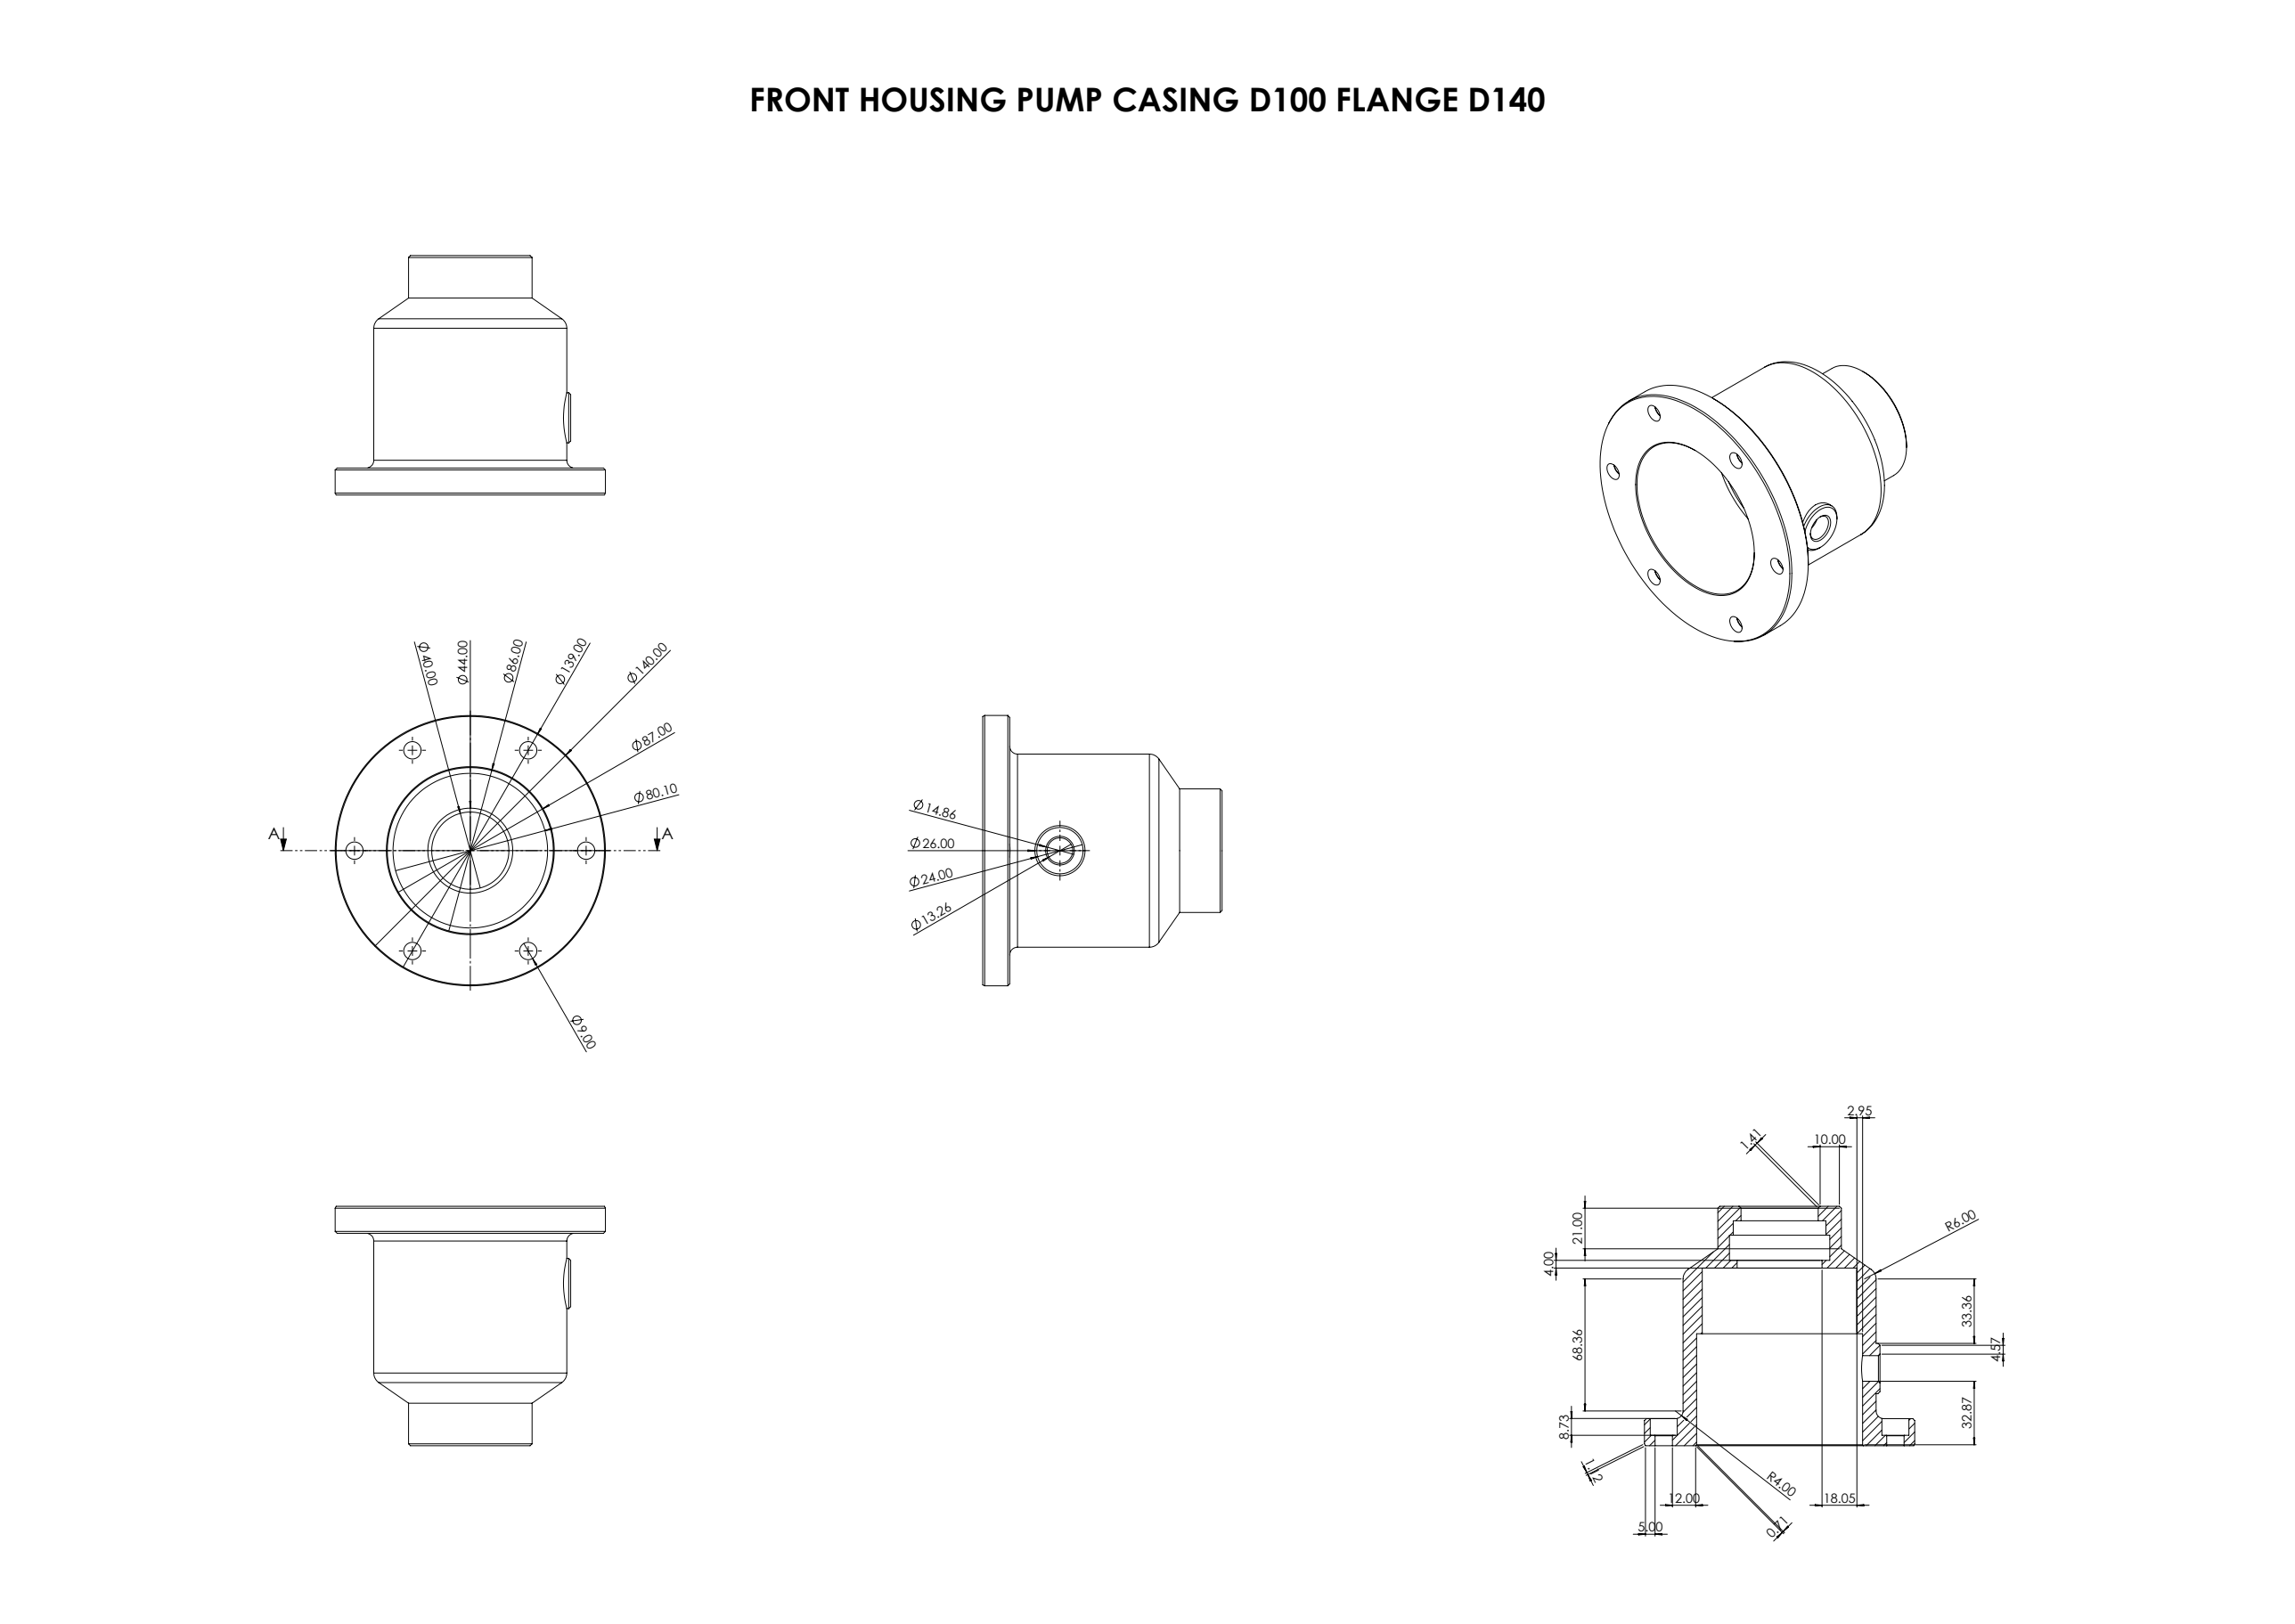
ISO-10303-21;
HEADER;
/* Generated by software containing ST-Developer
 * from STEP Tools, Inc. (www.steptools.com) 
 */

FILE_DESCRIPTION(
/* description */ (''),
/* implementation_level */ '2;1');

FILE_NAME(
/* name */ '01_Front_Housing_Pump_Casing_D100_Flange_D140.step',
/* time_stamp */ '2026-10-23T00:52:27+05:00',
/* author */ (''),
/* organization */ (''),
/* preprocessor_version */ 'ST-DEVELOPER v20.2',
/* originating_system */ 'Autodesk Translation Framework v15.15.0.0',
/* authorisation */ '');

FILE_SCHEMA (('AUTOMOTIVE_DESIGN { 1 0 10303 214 3 1 1 }'));
ENDSEC;

DATA;
#10=MECHANICAL_DESIGN_GEOMETRIC_PRESENTATION_REPRESENTATION('',(#1558,#1559,#1560,#1561,#1562,#1563,#1564),#59204);
#310=TOROIDAL_SURFACE('',#23784,5.4,0.4);
#311=TOROIDAL_SURFACE('',#23834,4.4,0.6);
#692=B_SPLINE_CURVE_WITH_KNOTS('',3,(#42442,#42443,#42444,#42445,#42446,
#42447,#42448,#42449,#42450,#42451,#42452,#42453,#42454,#42455,#42456,#42457),
 .UNSPECIFIED.,.F.,.F.,(4,2,2,2,2,2,2,4),(-0.827444006878981,-0.709137715093229,
-0.606258454477036,-0.552969769025734,-0.51054365769559,-0.463186805002842,
-0.385864633040324,-0.216479568668788),.UNSPECIFIED.);
#693=B_SPLINE_CURVE_WITH_KNOTS('',3,(#42466,#42467,#42468,#42469,#42470,
#42471,#42472,#42473,#42474,#42475),.UNSPECIFIED.,.F.,.F.,(4,2,2,2,4),(-0.52479568404363,
-0.512334893121172,-0.461457866065132,-0.380752711923638,-0.216468504749557),
 .UNSPECIFIED.);
#694=B_SPLINE_CURVE_WITH_KNOTS('',3,(#42479,#42480,#42481,#42482,#42483,
#42484,#42485,#42486,#42487,#42488,#42489,#42490,#42491,#42492,#42493,#42494),
 .UNSPECIFIED.,.F.,.F.,(4,2,2,2,2,2,2,4),(-0.827444006877975,-0.709137715092587,
-0.606258454476783,-0.552969769025578,-0.510543657695527,-0.463186805002854,
-0.385864633040295,-0.216479568668763),.UNSPECIFIED.);
#695=B_SPLINE_CURVE_WITH_KNOTS('',3,(#42498,#42499,#42500,#42501,#42502,
#42503,#42504,#42505,#42506,#42507,#42508,#42509,#42510,#42511,#42512,#42513),
 .UNSPECIFIED.,.F.,.F.,(4,2,2,2,2,2,2,4),(-0.827444006878145,-0.709137715092748,
-0.606258454476905,-0.552969769025703,-0.510543657695638,-0.463186805002939,
-0.385864633040348,-0.21647956866881),.UNSPECIFIED.);
#696=B_SPLINE_CURVE_WITH_KNOTS('',3,(#42517,#42518,#42519,#42520,#42521,
#42522,#42523,#42524,#42525,#42526),.UNSPECIFIED.,.F.,.F.,(4,2,2,2,4),(-0.828799355587065,
-0.7357048796955,-0.618324369294947,-0.558811967132771,-0.524795684044317),
 .UNSPECIFIED.);
#697=B_SPLINE_CURVE_WITH_KNOTS('',3,(#42528,#42529,#42530,#42531,#42532,
#42533,#42534,#42535,#42536,#42537),.UNSPECIFIED.,.F.,.F.,(4,2,2,2,4),(-0.524795684044317,
-0.512334893121834,-0.461457866065708,-0.380752711924124,-0.216468504749763),
 .UNSPECIFIED.);
#698=B_SPLINE_CURVE_WITH_KNOTS('',3,(#42542,#42543,#42544,#42545,#42546,
#42547,#42548,#42549,#42550,#42551,#42552,#42553,#42554,#42555,#42556,#42557),
 .UNSPECIFIED.,.F.,.F.,(4,2,2,2,2,2,2,4),(-0.827444006877793,-0.709137715092454,
-0.606258454476639,-0.552969769025454,-0.510543657695402,-0.463186805002724,
-0.385864633040191,-0.216479568668727),.UNSPECIFIED.);
#699=B_SPLINE_CURVE_WITH_KNOTS('',3,(#42560,#42561,#42562,#42563,#42564,
#42565,#42566,#42567,#42568,#42569),.UNSPECIFIED.,.F.,.F.,(4,2,2,2,4),(-0.828799355585381,
-0.735704879694107,-0.618324369293949,-0.558811967131987,-0.52479568404363),
 .UNSPECIFIED.);
#700=B_SPLINE_CURVE_WITH_KNOTS('',3,(#42606,#42607,#42608,#42609,#42610,
#42611,#42612,#42613,#42614,#42615),.UNSPECIFIED.,.F.,.F.,(4,2,2,2,4),(0.,
0.250118116648096,0.500236233296193,0.750349479868711,1.00046272644123),
 .UNSPECIFIED.);
#701=B_SPLINE_CURVE_WITH_KNOTS('',3,(#42616,#42617,#42618,#42619,#42620,
#42621,#42622,#42623,#42624,#42625,#42626,#42627,#42628,#42629,#42630,#42631,
#42632,#42633,#42634,#42635,#42636,#42637,#42638,#42639,#42640,#42641),
 .UNSPECIFIED.,.F.,.F.,(4,2,2,2,2,2,2,2,2,2,2,2,4),(1.00046272644123,1.25057597301375,
1.50068921958627,1.75080733623436,2.00092545288246,2.25104356953056,2.50116168617865,
2.75127493275117,3.00138817932369,3.25150142589621,3.50161467246873,3.75173278911682,
4.00185090576492),.UNSPECIFIED.);
#702=B_SPLINE_CURVE_WITH_KNOTS('',3,(#42653,#42654,#42655,#42656,#42657,
#42658,#42659,#42660,#42661,#42662,#42663,#42664,#42665,#42666,#42667,#42668,
#42669,#42670,#42671,#42672,#42673,#42674,#42675,#42676,#42677,#42678),
 .UNSPECIFIED.,.F.,.F.,(4,2,2,2,2,2,2,2,2,2,2,2,4),(0.,0.492179153056542,
0.984358306113084,1.47645655199157,1.96855479787006,2.46065304374855,2.95275128962704,
3.44493044268358,3.93710959574012,4.42928874879666,4.92146790185321,5.41356614773169,
5.90566439361018),.UNSPECIFIED.);
#703=B_SPLINE_CURVE_WITH_KNOTS('',3,(#42679,#42680,#42681,#42682,#42683,
#42684,#42685,#42686,#42687,#42688),.UNSPECIFIED.,.F.,.F.,(4,2,2,2,4),(5.90566439361018,
6.39776263948867,6.88986088536716,7.3820400384237,7.87421919148024),
 .UNSPECIFIED.);
#1518=SHAPE_REPRESENTATION_RELATIONSHIP('SRR','None',#59307,#1538);
#1538=ADVANCED_BREP_SHAPE_REPRESENTATION('',(#1585),#59194);
#1558=STYLED_ITEM('',(#59565),#21883);
#1559=STYLED_ITEM('',(#59565),#21884);
#1560=STYLED_ITEM('',(#59565),#21885);
#1561=STYLED_ITEM('',(#59565),#21908);
#1562=STYLED_ITEM('',(#59565),#21911);
#1563=STYLED_ITEM('',(#59565),#21915);
#1564=STYLED_ITEM('',(#59565),#1585);
#1585=MANIFOLD_SOLID_BREP('Front housing',#22814);
#1670=FACE_BOUND('',#4431,.T.);
#1671=FACE_BOUND('',#4435,.T.);
#1672=FACE_BOUND('',#4439,.T.);
#1673=FACE_BOUND('',#4443,.T.);
#1674=FACE_BOUND('',#4447,.T.);
#1675=FACE_BOUND('',#4451,.T.);
#1676=FACE_BOUND('',#4457,.T.);
#1677=FACE_BOUND('',#4465,.T.);
#1678=FACE_BOUND('',#4470,.T.);
#1679=FACE_BOUND('',#4471,.T.);
#1680=FACE_BOUND('',#4472,.T.);
#1681=FACE_BOUND('',#4473,.T.);
#1682=FACE_BOUND('',#4474,.T.);
#1683=FACE_BOUND('',#4475,.T.);
#1684=FACE_BOUND('',#4476,.T.);
#1685=FACE_BOUND('',#4478,.T.);
#1686=FACE_BOUND('',#4482,.T.);
#1687=FACE_BOUND('',#4483,.T.);
#1688=FACE_BOUND('',#4486,.T.);
#1689=FACE_BOUND('',#4494,.T.);
#1690=FACE_BOUND('',#4497,.T.);
#1691=FACE_BOUND('',#4500,.T.);
#1692=FACE_BOUND('',#4503,.T.);
#1693=FACE_BOUND('',#4506,.T.);
#2020=PLANE('',#23721);
#2021=PLANE('',#23722);
#2022=PLANE('',#23723);
#2023=PLANE('',#23724);
#2024=PLANE('',#23728);
#2025=PLANE('',#23732);
#2026=PLANE('',#23737);
#2027=PLANE('',#23745);
#2028=PLANE('',#23753);
#2029=PLANE('',#23761);
#2030=PLANE('',#23769);
#2031=PLANE('',#23777);
#2032=PLANE('',#23796);
#2033=PLANE('',#23813);
#2034=PLANE('',#23822);
#2035=PLANE('',#23832);
#2036=PLANE('',#23849);
#2037=PLANE('',#23853);
#2038=PLANE('',#23857);
#2039=PLANE('',#23861);
#2040=PLANE('',#23865);
#2504=CYLINDRICAL_SURFACE('',#23725,2.56);
#2505=CYLINDRICAL_SURFACE('',#23729,2.84);
#2506=CYLINDRICAL_SURFACE('',#23739,0.45);
#2507=CYLINDRICAL_SURFACE('',#23747,0.45);
#2508=CYLINDRICAL_SURFACE('',#23755,0.45);
#2509=CYLINDRICAL_SURFACE('',#23763,0.45);
#2510=CYLINDRICAL_SURFACE('',#23771,0.45);
#2511=CYLINDRICAL_SURFACE('',#23779,0.45);
#2512=CYLINDRICAL_SURFACE('',#23781,0.7);
#2513=CYLINDRICAL_SURFACE('',#23793,0.7);
#2514=CYLINDRICAL_SURFACE('',#23805,0.7);
#2515=CYLINDRICAL_SURFACE('',#23806,0.7);
#2516=CYLINDRICAL_SURFACE('',#23807,0.7);
#2517=CYLINDRICAL_SURFACE('',#23808,0.7);
#2518=CYLINDRICAL_SURFACE('',#23812,0.66285);
#2519=CYLINDRICAL_SURFACE('',#23817,1.3);
#2520=CYLINDRICAL_SURFACE('',#23824,4.3);
#2521=CYLINDRICAL_SURFACE('',#23830,2.);
#2522=CYLINDRICAL_SURFACE('',#23838,5.);
#2523=CYLINDRICAL_SURFACE('',#23843,3.2);
#2524=CYLINDRICAL_SURFACE('',#23846,7.);
#2525=CYLINDRICAL_SURFACE('',#23851,4.005);
#2526=CYLINDRICAL_SURFACE('',#23855,2.2);
#2527=CYLINDRICAL_SURFACE('',#23859,2.6);
#2528=CYLINDRICAL_SURFACE('',#23863,2.4);
#3045=FACE_OUTER_BOUND('',#4421,.T.);
#3046=FACE_OUTER_BOUND('',#4422,.T.);
#3047=FACE_OUTER_BOUND('',#4423,.T.);
#3048=FACE_OUTER_BOUND('',#4424,.T.);
#3049=FACE_OUTER_BOUND('',#4425,.T.);
#3050=FACE_OUTER_BOUND('',#4426,.T.);
#3051=FACE_OUTER_BOUND('',#4427,.T.);
#3052=FACE_OUTER_BOUND('',#4428,.T.);
#3053=FACE_OUTER_BOUND('',#4429,.T.);
#3054=FACE_OUTER_BOUND('',#4430,.T.);
#3055=FACE_OUTER_BOUND('',#4432,.T.);
#3056=FACE_OUTER_BOUND('',#4433,.T.);
#3057=FACE_OUTER_BOUND('',#4434,.T.);
#3058=FACE_OUTER_BOUND('',#4436,.T.);
#3059=FACE_OUTER_BOUND('',#4437,.T.);
#3060=FACE_OUTER_BOUND('',#4438,.T.);
#3061=FACE_OUTER_BOUND('',#4440,.T.);
#3062=FACE_OUTER_BOUND('',#4441,.T.);
#3063=FACE_OUTER_BOUND('',#4442,.T.);
#3064=FACE_OUTER_BOUND('',#4444,.T.);
#3065=FACE_OUTER_BOUND('',#4445,.T.);
#3066=FACE_OUTER_BOUND('',#4446,.T.);
#3067=FACE_OUTER_BOUND('',#4448,.T.);
#3068=FACE_OUTER_BOUND('',#4449,.T.);
#3069=FACE_OUTER_BOUND('',#4450,.T.);
#3070=FACE_OUTER_BOUND('',#4452,.T.);
#3071=FACE_OUTER_BOUND('',#4453,.T.);
#3072=FACE_OUTER_BOUND('',#4454,.T.);
#3073=FACE_OUTER_BOUND('',#4455,.T.);
#3074=FACE_OUTER_BOUND('',#4456,.T.);
#3075=FACE_OUTER_BOUND('',#4458,.T.);
#3076=FACE_OUTER_BOUND('',#4459,.T.);
#3077=FACE_OUTER_BOUND('',#4460,.T.);
#3078=FACE_OUTER_BOUND('',#4461,.T.);
#3079=FACE_OUTER_BOUND('',#4462,.T.);
#3080=FACE_OUTER_BOUND('',#4463,.T.);
#3081=FACE_OUTER_BOUND('',#4464,.T.);
#3082=FACE_OUTER_BOUND('',#4466,.T.);
#3083=FACE_OUTER_BOUND('',#4467,.T.);
#3084=FACE_OUTER_BOUND('',#4468,.T.);
#3085=FACE_OUTER_BOUND('',#4469,.T.);
#3086=FACE_OUTER_BOUND('',#4477,.T.);
#3087=FACE_OUTER_BOUND('',#4479,.T.);
#3088=FACE_OUTER_BOUND('',#4480,.T.);
#3089=FACE_OUTER_BOUND('',#4481,.T.);
#3090=FACE_OUTER_BOUND('',#4484,.T.);
#3091=FACE_OUTER_BOUND('',#4485,.T.);
#3092=FACE_OUTER_BOUND('',#4487,.T.);
#3093=FACE_OUTER_BOUND('',#4488,.T.);
#3094=FACE_OUTER_BOUND('',#4489,.T.);
#3095=FACE_OUTER_BOUND('',#4490,.T.);
#3096=FACE_OUTER_BOUND('',#4491,.T.);
#3097=FACE_OUTER_BOUND('',#4492,.T.);
#3098=FACE_OUTER_BOUND('',#4493,.T.);
#3099=FACE_OUTER_BOUND('',#4495,.T.);
#3100=FACE_OUTER_BOUND('',#4496,.T.);
#3101=FACE_OUTER_BOUND('',#4498,.T.);
#3102=FACE_OUTER_BOUND('',#4499,.T.);
#3103=FACE_OUTER_BOUND('',#4501,.T.);
#3104=FACE_OUTER_BOUND('',#4502,.T.);
#3105=FACE_OUTER_BOUND('',#4504,.T.);
#3106=FACE_OUTER_BOUND('',#4505,.T.);
#4421=EDGE_LOOP('',(#16438,#16439,#16440,#16441));
#4422=EDGE_LOOP('',(#16442,#16443,#16444,#16445));
#4423=EDGE_LOOP('',(#16446,#16447,#16448,#16449));
#4424=EDGE_LOOP('',(#16450,#16451,#16452,#16453));
#4425=EDGE_LOOP('',(#16454,#16455,#16456,#16457));
#4426=EDGE_LOOP('',(#16458,#16459,#16460,#16461));
#4427=EDGE_LOOP('',(#16462,#16463,#16464,#16465));
#4428=EDGE_LOOP('',(#16466,#16467,#16468,#16469,#16470,#16471,#16472));
#4429=EDGE_LOOP('',(#16473,#16474,#16475,#16476,#16477));
#4430=EDGE_LOOP('',(#16478));
#4431=EDGE_LOOP('',(#16479));
#4432=EDGE_LOOP('',(#16480,#16481,#16482,#16483,#16484));
#4433=EDGE_LOOP('',(#16485,#16486,#16487,#16488,#16489));
#4434=EDGE_LOOP('',(#16490));
#4435=EDGE_LOOP('',(#16491));
#4436=EDGE_LOOP('',(#16492,#16493,#16494,#16495,#16496));
#4437=EDGE_LOOP('',(#16497,#16498,#16499,#16500,#16501));
#4438=EDGE_LOOP('',(#16502));
#4439=EDGE_LOOP('',(#16503));
#4440=EDGE_LOOP('',(#16504,#16505,#16506,#16507,#16508));
#4441=EDGE_LOOP('',(#16509,#16510,#16511,#16512,#16513));
#4442=EDGE_LOOP('',(#16514));
#4443=EDGE_LOOP('',(#16515));
#4444=EDGE_LOOP('',(#16516,#16517,#16518,#16519,#16520));
#4445=EDGE_LOOP('',(#16521,#16522,#16523,#16524,#16525));
#4446=EDGE_LOOP('',(#16526));
#4447=EDGE_LOOP('',(#16527));
#4448=EDGE_LOOP('',(#16528,#16529,#16530,#16531,#16532));
#4449=EDGE_LOOP('',(#16533,#16534,#16535,#16536,#16537));
#4450=EDGE_LOOP('',(#16538));
#4451=EDGE_LOOP('',(#16539));
#4452=EDGE_LOOP('',(#16540,#16541,#16542,#16543,#16544));
#4453=EDGE_LOOP('',(#16545,#16546,#16547,#16548,#16549,#16550));
#4454=EDGE_LOOP('',(#16551,#16552,#16553,#16554,#16555,#16556,#16557,#16558,
#16559,#16560,#16561,#16562,#16563,#16564,#16565,#16566,#16567));
#4455=EDGE_LOOP('',(#16568,#16569,#16570,#16571,#16572,#16573));
#4456=EDGE_LOOP('',(#16574));
#4457=EDGE_LOOP('',(#16575,#16576,#16577,#16578,#16579,#16580,#16581,#16582,
#16583,#16584,#16585,#16586,#16587,#16588,#16589,#16590,#16591));
#4458=EDGE_LOOP('',(#16592,#16593,#16594,#16595,#16596,#16597,#16598));
#4459=EDGE_LOOP('',(#16599,#16600,#16601,#16602,#16603,#16604));
#4460=EDGE_LOOP('',(#16605,#16606,#16607,#16608,#16609,#16610));
#4461=EDGE_LOOP('',(#16611,#16612,#16613,#16614,#16615,#16616));
#4462=EDGE_LOOP('',(#16617,#16618,#16619,#16620));
#4463=EDGE_LOOP('',(#16621,#16622,#16623,#16624,#16625));
#4464=EDGE_LOOP('',(#16626));
#4465=EDGE_LOOP('',(#16627));
#4466=EDGE_LOOP('',(#16628,#16629,#16630,#16631));
#4467=EDGE_LOOP('',(#16632,#16633,#16634,#16635,#16636));
#4468=EDGE_LOOP('',(#16637,#16638,#16639,#16640,#16641));
#4469=EDGE_LOOP('',(#16642));
#4470=EDGE_LOOP('',(#16643));
#4471=EDGE_LOOP('',(#16644));
#4472=EDGE_LOOP('',(#16645));
#4473=EDGE_LOOP('',(#16646));
#4474=EDGE_LOOP('',(#16647));
#4475=EDGE_LOOP('',(#16648));
#4476=EDGE_LOOP('',(#16649));
#4477=EDGE_LOOP('',(#16650,#16651,#16652,#16653,#16654));
#4478=EDGE_LOOP('',(#16655,#16656));
#4479=EDGE_LOOP('',(#16657,#16658,#16659,#16660,#16661));
#4480=EDGE_LOOP('',(#16662,#16663,#16664,#16665,#16666));
#4481=EDGE_LOOP('',(#16667));
#4482=EDGE_LOOP('',(#16668,#16669,#16670,#16671,#16672,#16673,#16674));
#4483=EDGE_LOOP('',(#16675));
#4484=EDGE_LOOP('',(#16676,#16677,#16678,#16679));
#4485=EDGE_LOOP('',(#16680,#16681,#16682,#16683));
#4486=EDGE_LOOP('',(#16684,#16685));
#4487=EDGE_LOOP('',(#16686,#16687,#16688,#16689));
#4488=EDGE_LOOP('',(#16690,#16691,#16692,#16693));
#4489=EDGE_LOOP('',(#16694,#16695,#16696,#16697));
#4490=EDGE_LOOP('',(#16698,#16699,#16700,#16701));
#4491=EDGE_LOOP('',(#16702,#16703,#16704,#16705));
#4492=EDGE_LOOP('',(#16706,#16707,#16708,#16709));
#4493=EDGE_LOOP('',(#16710));
#4494=EDGE_LOOP('',(#16711));
#4495=EDGE_LOOP('',(#16712,#16713,#16714,#16715));
#4496=EDGE_LOOP('',(#16716));
#4497=EDGE_LOOP('',(#16717));
#4498=EDGE_LOOP('',(#16718,#16719,#16720,#16721));
#4499=EDGE_LOOP('',(#16722));
#4500=EDGE_LOOP('',(#16723));
#4501=EDGE_LOOP('',(#16724,#16725,#16726,#16727));
#4502=EDGE_LOOP('',(#16728));
#4503=EDGE_LOOP('',(#16729));
#4504=EDGE_LOOP('',(#16730,#16731,#16732,#16733));
#4505=EDGE_LOOP('',(#16734));
#4506=EDGE_LOOP('',(#16735));
#5919=LINE('',#42307,#7352);
#5920=LINE('',#42309,#7353);
#5921=LINE('',#42311,#7354);
#5922=LINE('',#42312,#7355);
#5923=LINE('',#42315,#7356);
#5924=LINE('',#42317,#7357);
#5925=LINE('',#42318,#7358);
#5926=LINE('',#42321,#7359);
#5927=LINE('',#42323,#7360);
#5928=LINE('',#42324,#7361);
#5929=LINE('',#42327,#7362);
#5930=LINE('',#42329,#7363);
#5931=LINE('',#42330,#7364);
#5932=LINE('',#42335,#7365);
#5933=LINE('',#42339,#7366);
#5934=LINE('',#42341,#7367);
#5935=LINE('',#42342,#7368);
#5936=LINE('',#42351,#7369);
#5937=LINE('',#42360,#7370);
#5938=LINE('',#42366,#7371);
#5939=LINE('',#42375,#7372);
#5940=LINE('',#42381,#7373);
#5941=LINE('',#42390,#7374);
#5942=LINE('',#42396,#7375);
#5943=LINE('',#42405,#7376);
#5944=LINE('',#42411,#7377);
#5945=LINE('',#42420,#7378);
#5946=LINE('',#42426,#7379);
#5947=LINE('',#42435,#7380);
#5948=LINE('',#42459,#7381);
#5949=LINE('',#42573,#7382);
#5950=LINE('',#42589,#7383);
#5951=LINE('',#42591,#7384);
#5952=LINE('',#42593,#7385);
#5953=LINE('',#42595,#7386);
#5954=LINE('',#42600,#7387);
#5955=LINE('',#42604,#7388);
#5956=LINE('',#42647,#7389);
#5957=LINE('',#42651,#7390);
#5958=LINE('',#42695,#7391);
#5959=LINE('',#42702,#7392);
#5960=LINE('',#42708,#7393);
#5961=LINE('',#42715,#7394);
#5962=LINE('',#42726,#7395);
#5963=LINE('',#42729,#7396);
#5964=LINE('',#42734,#7397);
#5965=LINE('',#42736,#7398);
#5966=LINE('',#42740,#7399);
#5967=LINE('',#42744,#7400);
#5968=LINE('',#42746,#7401);
#5969=LINE('',#42752,#7402);
#5970=LINE('',#42759,#7403);
#5971=LINE('',#42766,#7404);
#5972=LINE('',#42773,#7405);
#7352=VECTOR('',#26899,1.);
#7353=VECTOR('',#26900,1.);
#7354=VECTOR('',#26901,1.);
#7355=VECTOR('',#26902,1.);
#7356=VECTOR('',#26905,1.);
#7357=VECTOR('',#26906,1.);
#7358=VECTOR('',#26907,1.);
#7359=VECTOR('',#26910,1.);
#7360=VECTOR('',#26911,1.);
#7361=VECTOR('',#26912,1.);
#7362=VECTOR('',#26915,1.);
#7363=VECTOR('',#26916,1.);
#7364=VECTOR('',#26917,1.);
#7365=VECTOR('',#26922,1.);
#7366=VECTOR('',#26927,1.);
#7367=VECTOR('',#26928,1.);
#7368=VECTOR('',#26929,1.);
#7369=VECTOR('',#26942,0.4625);
#7370=VECTOR('',#26953,0.45);
#7371=VECTOR('',#26960,0.4625);
#7372=VECTOR('',#26971,0.45);
#7373=VECTOR('',#26978,0.4625);
#7374=VECTOR('',#26989,0.45);
#7375=VECTOR('',#26996,0.4625);
#7376=VECTOR('',#27007,0.45);
#7377=VECTOR('',#27014,0.4625);
#7378=VECTOR('',#27025,0.45);
#7379=VECTOR('',#27032,0.4625);
#7380=VECTOR('',#27043,0.45);
#7381=VECTOR('',#27052,0.7);
#7382=VECTOR('',#27075,0.7);
#7383=VECTOR('',#27098,0.7);
#7384=VECTOR('',#27101,0.7);
#7385=VECTOR('',#27104,0.7);
#7386=VECTOR('',#27107,0.7);
#7387=VECTOR('',#27112,0.70285);
#7388=VECTOR('',#27117,0.66285);
#7389=VECTOR('',#27124,1.25);
#7390=VECTOR('',#27129,1.3);
#7391=VECTOR('',#27136,4.325);
#7392=VECTOR('',#27145,4.3);
#7393=VECTOR('',#27152,2.05);
#7394=VECTOR('',#27161,2.);
#7395=VECTOR('',#27176,5.);
#7396=VECTOR('',#27179,4.1);
#7397=VECTOR('',#27186,3.15);
#7398=VECTOR('',#27189,3.2);
#7399=VECTOR('',#27194,6.95);
#7400=VECTOR('',#27199,7.);
#7401=VECTOR('',#27202,6.975);
#7402=VECTOR('',#27209,4.005);
#7403=VECTOR('',#27218,2.2);
#7404=VECTOR('',#27227,2.6);
#7405=VECTOR('',#27236,2.4);
#8662=CIRCLE('',#23726,2.56);
#8663=CIRCLE('',#23727,2.56);
#8664=CIRCLE('',#23730,2.84);
#8665=CIRCLE('',#23731,2.84);
#8666=CIRCLE('',#23734,0.475000000000001);
#8667=CIRCLE('',#23735,0.45);
#8668=CIRCLE('',#23736,0.45);
#8669=CIRCLE('',#23738,0.7);
#8670=CIRCLE('',#23740,0.45);
#8671=CIRCLE('',#23742,0.475);
#8672=CIRCLE('',#23743,0.45);
#8673=CIRCLE('',#23744,0.45);
#8674=CIRCLE('',#23746,0.7);
#8675=CIRCLE('',#23748,0.45);
#8676=CIRCLE('',#23750,0.475);
#8677=CIRCLE('',#23751,0.45);
#8678=CIRCLE('',#23752,0.45);
#8679=CIRCLE('',#23754,0.7);
#8680=CIRCLE('',#23756,0.45);
#8681=CIRCLE('',#23758,0.475000000000001);
#8682=CIRCLE('',#23759,0.45);
#8683=CIRCLE('',#23760,0.45);
#8684=CIRCLE('',#23762,0.7);
#8685=CIRCLE('',#23764,0.45);
#8686=CIRCLE('',#23766,0.475);
#8687=CIRCLE('',#23767,0.45);
#8688=CIRCLE('',#23768,0.45);
#8689=CIRCLE('',#23770,0.7);
#8690=CIRCLE('',#23772,0.45);
#8691=CIRCLE('',#23774,0.475);
#8692=CIRCLE('',#23775,0.45);
#8693=CIRCLE('',#23776,0.45);
#8694=CIRCLE('',#23778,0.7);
#8695=CIRCLE('',#23780,0.45);
#8696=CIRCLE('',#23782,0.7);
#8697=CIRCLE('',#23783,0.7);
#8698=CIRCLE('',#23785,5.);
#8699=CIRCLE('',#23786,0.4);
#8700=CIRCLE('',#23787,5.4);
#8701=CIRCLE('',#23788,5.4);
#8702=CIRCLE('',#23789,5.4);
#8703=CIRCLE('',#23790,5.4);
#8704=CIRCLE('',#23791,5.4);
#8705=CIRCLE('',#23792,5.4);
#8706=CIRCLE('',#23794,0.7);
#8707=CIRCLE('',#23795,0.7);
#8708=CIRCLE('',#23797,6.9);
#8709=CIRCLE('',#23798,0.7);
#8710=CIRCLE('',#23799,0.7);
#8711=CIRCLE('',#23800,0.7);
#8712=CIRCLE('',#23801,0.7);
#8713=CIRCLE('',#23802,0.7);
#8714=CIRCLE('',#23803,0.7);
#8715=CIRCLE('',#23804,0.7);
#8716=CIRCLE('',#23810,0.74285);
#8717=CIRCLE('',#23811,0.66285);
#8718=CIRCLE('',#23814,1.2);
#8719=CIRCLE('',#23816,1.3);
#8720=CIRCLE('',#23819,4.3);
#8721=CIRCLE('',#23820,4.3);
#8722=CIRCLE('',#23821,4.35);
#8723=CIRCLE('',#23823,6.95);
#8724=CIRCLE('',#23825,4.3);
#8725=CIRCLE('',#23827,2.1);
#8726=CIRCLE('',#23828,2.);
#8727=CIRCLE('',#23829,2.);
#8728=CIRCLE('',#23831,2.);
#8729=CIRCLE('',#23833,3.1);
#8730=CIRCLE('',#23835,5.);
#8731=CIRCLE('',#23836,0.6);
#8732=CIRCLE('',#23837,4.74223748569721);
#8733=CIRCLE('',#23840,3.2);
#8734=CIRCLE('',#23842,3.2);
#8735=CIRCLE('',#23845,7.);
#8736=CIRCLE('',#23847,7.);
#8737=CIRCLE('',#23850,4.005);
#8738=CIRCLE('',#23852,4.005);
#8739=CIRCLE('',#23854,2.2);
#8740=CIRCLE('',#23856,2.2);
#8741=CIRCLE('',#23858,2.6);
#8742=CIRCLE('',#23860,2.6);
#8743=CIRCLE('',#23862,2.4);
#8744=CIRCLE('',#23864,2.4);
#9749=VERTEX_POINT('',#42305);
#9750=VERTEX_POINT('',#42306);
#9751=VERTEX_POINT('',#42308);
#9752=VERTEX_POINT('',#42310);
#9753=VERTEX_POINT('',#42314);
#9754=VERTEX_POINT('',#42316);
#9755=VERTEX_POINT('',#42320);
#9756=VERTEX_POINT('',#42322);
#9757=VERTEX_POINT('',#42326);
#9758=VERTEX_POINT('',#42328);
#9759=VERTEX_POINT('',#42332);
#9760=VERTEX_POINT('',#42334);
#9761=VERTEX_POINT('',#42338);
#9762=VERTEX_POINT('',#42340);
#9763=VERTEX_POINT('',#42348);
#9764=VERTEX_POINT('',#42350);
#9765=VERTEX_POINT('',#42352);
#9766=VERTEX_POINT('',#42356);
#9767=VERTEX_POINT('',#42359);
#9768=VERTEX_POINT('',#42363);
#9769=VERTEX_POINT('',#42365);
#9770=VERTEX_POINT('',#42367);
#9771=VERTEX_POINT('',#42371);
#9772=VERTEX_POINT('',#42374);
#9773=VERTEX_POINT('',#42378);
#9774=VERTEX_POINT('',#42380);
#9775=VERTEX_POINT('',#42382);
#9776=VERTEX_POINT('',#42386);
#9777=VERTEX_POINT('',#42389);
#9778=VERTEX_POINT('',#42393);
#9779=VERTEX_POINT('',#42395);
#9780=VERTEX_POINT('',#42397);
#9781=VERTEX_POINT('',#42401);
#9782=VERTEX_POINT('',#42404);
#9783=VERTEX_POINT('',#42408);
#9784=VERTEX_POINT('',#42410);
#9785=VERTEX_POINT('',#42412);
#9786=VERTEX_POINT('',#42416);
#9787=VERTEX_POINT('',#42419);
#9788=VERTEX_POINT('',#42423);
#9789=VERTEX_POINT('',#42425);
#9790=VERTEX_POINT('',#42427);
#9791=VERTEX_POINT('',#42431);
#9792=VERTEX_POINT('',#42434);
#9793=VERTEX_POINT('',#42438);
#9794=VERTEX_POINT('',#42439);
#9795=VERTEX_POINT('',#42441);
#9796=VERTEX_POINT('',#42461);
#9797=VERTEX_POINT('',#42463);
#9798=VERTEX_POINT('',#42465);
#9799=VERTEX_POINT('',#42476);
#9800=VERTEX_POINT('',#42478);
#9801=VERTEX_POINT('',#42495);
#9802=VERTEX_POINT('',#42497);
#9803=VERTEX_POINT('',#42514);
#9804=VERTEX_POINT('',#42516);
#9805=VERTEX_POINT('',#42527);
#9806=VERTEX_POINT('',#42539);
#9807=VERTEX_POINT('',#42541);
#9808=VERTEX_POINT('',#42558);
#9809=VERTEX_POINT('',#42571);
#9810=VERTEX_POINT('',#42576);
#9811=VERTEX_POINT('',#42579);
#9812=VERTEX_POINT('',#42582);
#9813=VERTEX_POINT('',#42585);
#9814=VERTEX_POINT('',#42597);
#9815=VERTEX_POINT('',#42599);
#9816=VERTEX_POINT('',#42603);
#9817=VERTEX_POINT('',#42605);
#9818=VERTEX_POINT('',#42643);
#9819=VERTEX_POINT('',#42646);
#9820=VERTEX_POINT('',#42650);
#9821=VERTEX_POINT('',#42652);
#9822=VERTEX_POINT('',#42690);
#9823=VERTEX_POINT('',#42691);
#9824=VERTEX_POINT('',#42694);
#9825=VERTEX_POINT('',#42698);
#9826=VERTEX_POINT('',#42701);
#9827=VERTEX_POINT('',#42705);
#9828=VERTEX_POINT('',#42707);
#9829=VERTEX_POINT('',#42709);
#9830=VERTEX_POINT('',#42713);
#9831=VERTEX_POINT('',#42717);
#9832=VERTEX_POINT('',#42720);
#9833=VERTEX_POINT('',#42722);
#9834=VERTEX_POINT('',#42728);
#9835=VERTEX_POINT('',#42732);
#9836=VERTEX_POINT('',#42738);
#9837=VERTEX_POINT('',#42742);
#9838=VERTEX_POINT('',#42748);
#9839=VERTEX_POINT('',#42751);
#9840=VERTEX_POINT('',#42755);
#9841=VERTEX_POINT('',#42758);
#9842=VERTEX_POINT('',#42762);
#9843=VERTEX_POINT('',#42765);
#9844=VERTEX_POINT('',#42769);
#9845=VERTEX_POINT('',#42772);
#12223=EDGE_CURVE('',#9749,#9750,#5919,.T.);
#12224=EDGE_CURVE('',#9749,#9751,#5920,.T.);
#12225=EDGE_CURVE('',#9751,#9752,#5921,.T.);
#12226=EDGE_CURVE('',#9750,#9752,#5922,.T.);
#12227=EDGE_CURVE('',#9753,#9749,#5923,.T.);
#12228=EDGE_CURVE('',#9753,#9754,#5924,.T.);
#12229=EDGE_CURVE('',#9754,#9751,#5925,.T.);
#12230=EDGE_CURVE('',#9755,#9753,#5926,.T.);
#12231=EDGE_CURVE('',#9755,#9756,#5927,.T.);
#12232=EDGE_CURVE('',#9756,#9754,#5928,.T.);
#12233=EDGE_CURVE('',#9757,#9755,#5929,.T.);
#12234=EDGE_CURVE('',#9757,#9758,#5930,.T.);
#12235=EDGE_CURVE('',#9758,#9756,#5931,.T.);
#12236=EDGE_CURVE('',#9759,#9757,#8662,.T.);
#12237=EDGE_CURVE('',#9759,#9760,#5932,.T.);
#12238=EDGE_CURVE('',#9760,#9758,#8663,.T.);
#12239=EDGE_CURVE('',#9761,#9759,#5933,.T.);
#12240=EDGE_CURVE('',#9761,#9762,#5934,.T.);
#12241=EDGE_CURVE('',#9762,#9760,#5935,.T.);
#12242=EDGE_CURVE('',#9750,#9761,#8664,.T.);
#12243=EDGE_CURVE('',#9752,#9762,#8665,.T.);
#12244=EDGE_CURVE('',#9763,#9763,#8666,.T.);
#12245=EDGE_CURVE('',#9763,#9764,#5936,.T.);
#12246=EDGE_CURVE('',#9764,#9765,#8667,.T.);
#12247=EDGE_CURVE('',#9765,#9764,#8668,.T.);
#12248=EDGE_CURVE('',#9766,#9766,#8669,.T.);
#12249=EDGE_CURVE('',#9765,#9767,#5937,.T.);
#12250=EDGE_CURVE('',#9767,#9767,#8670,.T.);
#12251=EDGE_CURVE('',#9768,#9768,#8671,.T.);
#12252=EDGE_CURVE('',#9768,#9769,#5938,.T.);
#12253=EDGE_CURVE('',#9769,#9770,#8672,.T.);
#12254=EDGE_CURVE('',#9770,#9769,#8673,.T.);
#12255=EDGE_CURVE('',#9771,#9771,#8674,.T.);
#12256=EDGE_CURVE('',#9770,#9772,#5939,.T.);
#12257=EDGE_CURVE('',#9772,#9772,#8675,.T.);
#12258=EDGE_CURVE('',#9773,#9773,#8676,.T.);
#12259=EDGE_CURVE('',#9773,#9774,#5940,.T.);
#12260=EDGE_CURVE('',#9774,#9775,#8677,.T.);
#12261=EDGE_CURVE('',#9775,#9774,#8678,.T.);
#12262=EDGE_CURVE('',#9776,#9776,#8679,.T.);
#12263=EDGE_CURVE('',#9775,#9777,#5941,.T.);
#12264=EDGE_CURVE('',#9777,#9777,#8680,.T.);
#12265=EDGE_CURVE('',#9778,#9778,#8681,.T.);
#12266=EDGE_CURVE('',#9778,#9779,#5942,.T.);
#12267=EDGE_CURVE('',#9779,#9780,#8682,.T.);
#12268=EDGE_CURVE('',#9780,#9779,#8683,.T.);
#12269=EDGE_CURVE('',#9781,#9781,#8684,.T.);
#12270=EDGE_CURVE('',#9780,#9782,#5943,.T.);
#12271=EDGE_CURVE('',#9782,#9782,#8685,.T.);
#12272=EDGE_CURVE('',#9783,#9783,#8686,.T.);
#12273=EDGE_CURVE('',#9783,#9784,#5944,.T.);
#12274=EDGE_CURVE('',#9784,#9785,#8687,.T.);
#12275=EDGE_CURVE('',#9785,#9784,#8688,.T.);
#12276=EDGE_CURVE('',#9786,#9786,#8689,.T.);
#12277=EDGE_CURVE('',#9785,#9787,#5945,.T.);
#12278=EDGE_CURVE('',#9787,#9787,#8690,.T.);
#12279=EDGE_CURVE('',#9788,#9788,#8691,.T.);
#12280=EDGE_CURVE('',#9788,#9789,#5946,.T.);
#12281=EDGE_CURVE('',#9789,#9790,#8692,.T.);
#12282=EDGE_CURVE('',#9790,#9789,#8693,.T.);
#12283=EDGE_CURVE('',#9791,#9791,#8694,.T.);
#12284=EDGE_CURVE('',#9790,#9792,#5947,.T.);
#12285=EDGE_CURVE('',#9792,#9792,#8695,.T.);
#12286=EDGE_CURVE('',#9793,#9794,#8696,.T.);
#12287=EDGE_CURVE('',#9795,#9793,#692,.T.);
#12288=EDGE_CURVE('',#9794,#9795,#8697,.T.);
#12289=EDGE_CURVE('',#9794,#9791,#5948,.T.);
#12290=EDGE_CURVE('',#9796,#9796,#8698,.T.);
#12291=EDGE_CURVE('',#9796,#9797,#8699,.T.);
#12292=EDGE_CURVE('',#9797,#9798,#693,.T.);
#12293=EDGE_CURVE('',#9798,#9799,#8700,.T.);
#12294=EDGE_CURVE('',#9799,#9800,#694,.T.);
#12295=EDGE_CURVE('',#9800,#9801,#8701,.T.);
#12296=EDGE_CURVE('',#9801,#9802,#695,.T.);
#12297=EDGE_CURVE('',#9802,#9803,#8702,.T.);
#12298=EDGE_CURVE('',#9803,#9804,#696,.T.);
#12299=EDGE_CURVE('',#9804,#9805,#697,.T.);
#12300=EDGE_CURVE('',#9805,#9795,#8703,.T.);
#12301=EDGE_CURVE('',#9793,#9806,#8704,.T.);
#12302=EDGE_CURVE('',#9806,#9807,#698,.T.);
#12303=EDGE_CURVE('',#9807,#9808,#8705,.T.);
#12304=EDGE_CURVE('',#9808,#9797,#699,.T.);
#12305=EDGE_CURVE('',#9809,#9806,#8706,.T.);
#12306=EDGE_CURVE('',#9809,#9786,#5949,.T.);
#12307=EDGE_CURVE('',#9807,#9809,#8707,.T.);
#12308=EDGE_CURVE('',#9810,#9810,#8708,.T.);
#12309=EDGE_CURVE('',#9805,#9803,#8709,.T.);
#12310=EDGE_CURVE('',#9802,#9811,#8710,.T.);
#12311=EDGE_CURVE('',#9811,#9801,#8711,.T.);
#12312=EDGE_CURVE('',#9800,#9812,#8712,.T.);
#12313=EDGE_CURVE('',#9812,#9799,#8713,.T.);
#12314=EDGE_CURVE('',#9798,#9813,#8714,.T.);
#12315=EDGE_CURVE('',#9813,#9808,#8715,.T.);
#12316=EDGE_CURVE('',#9813,#9781,#5950,.T.);
#12317=EDGE_CURVE('',#9812,#9776,#5951,.T.);
#12318=EDGE_CURVE('',#9811,#9771,#5952,.T.);
#12319=EDGE_CURVE('',#9804,#9766,#5953,.T.);
#12320=EDGE_CURVE('',#9814,#9814,#8716,.T.);
#12321=EDGE_CURVE('',#9814,#9815,#5954,.T.);
#12322=EDGE_CURVE('',#9815,#9815,#8717,.T.);
#12323=EDGE_CURVE('',#9815,#9816,#5955,.T.);
#12324=EDGE_CURVE('',#9817,#9816,#700,.T.);
#12325=EDGE_CURVE('',#9816,#9817,#701,.T.);
#12326=EDGE_CURVE('',#9818,#9818,#8718,.T.);
#12327=EDGE_CURVE('',#9818,#9819,#5956,.T.);
#12328=EDGE_CURVE('',#9819,#9819,#8719,.T.);
#12329=EDGE_CURVE('',#9819,#9820,#5957,.T.);
#12330=EDGE_CURVE('',#9821,#9820,#702,.T.);
#12331=EDGE_CURVE('',#9820,#9821,#703,.T.);
#12332=EDGE_CURVE('',#9822,#9823,#8720,.T.);
#12333=EDGE_CURVE('',#9823,#9822,#8721,.T.);
#12334=EDGE_CURVE('',#9822,#9824,#5958,.T.);
#12335=EDGE_CURVE('',#9824,#9824,#8722,.T.);
#12336=EDGE_CURVE('',#9825,#9825,#8723,.T.);
#12337=EDGE_CURVE('',#9823,#9826,#5959,.T.);
#12338=EDGE_CURVE('',#9826,#9826,#8724,.T.);
#12339=EDGE_CURVE('',#9827,#9827,#8725,.T.);
#12340=EDGE_CURVE('',#9827,#9828,#5960,.T.);
#12341=EDGE_CURVE('',#9828,#9829,#8726,.T.);
#12342=EDGE_CURVE('',#9829,#9828,#8727,.T.);
#12343=EDGE_CURVE('',#9830,#9830,#8728,.T.);
#12344=EDGE_CURVE('',#9830,#9829,#5961,.T.);
#12345=EDGE_CURVE('',#9831,#9831,#8729,.T.);
#12346=EDGE_CURVE('',#9832,#9832,#8730,.T.);
#12347=EDGE_CURVE('',#9832,#9833,#8731,.T.);
#12348=EDGE_CURVE('',#9833,#9833,#8732,.T.);
#12349=EDGE_CURVE('',#9796,#9832,#5962,.T.);
#12350=EDGE_CURVE('',#9833,#9834,#5963,.T.);
#12351=EDGE_CURVE('',#9834,#9834,#8733,.T.);
#12352=EDGE_CURVE('',#9835,#9835,#8734,.T.);
#12353=EDGE_CURVE('',#9835,#9831,#5964,.T.);
#12354=EDGE_CURVE('',#9834,#9835,#5965,.T.);
#12355=EDGE_CURVE('',#9836,#9836,#8735,.T.);
#12356=EDGE_CURVE('',#9836,#9810,#5966,.T.);
#12357=EDGE_CURVE('',#9837,#9837,#8736,.T.);
#12358=EDGE_CURVE('',#9837,#9836,#5967,.T.);
#12359=EDGE_CURVE('',#9825,#9837,#5968,.T.);
#12360=EDGE_CURVE('',#9838,#9838,#8737,.T.);
#12361=EDGE_CURVE('',#9838,#9839,#5969,.T.);
#12362=EDGE_CURVE('',#9839,#9839,#8738,.T.);
#12363=EDGE_CURVE('',#9840,#9840,#8739,.T.);
#12364=EDGE_CURVE('',#9840,#9841,#5970,.T.);
#12365=EDGE_CURVE('',#9841,#9841,#8740,.T.);
#12366=EDGE_CURVE('',#9842,#9842,#8741,.T.);
#12367=EDGE_CURVE('',#9842,#9843,#5971,.T.);
#12368=EDGE_CURVE('',#9843,#9843,#8742,.T.);
#12369=EDGE_CURVE('',#9844,#9844,#8743,.T.);
#12370=EDGE_CURVE('',#9844,#9845,#5972,.T.);
#12371=EDGE_CURVE('',#9845,#9845,#8744,.T.);
#16438=ORIENTED_EDGE('',*,*,#12223,.F.);
#16439=ORIENTED_EDGE('',*,*,#12224,.T.);
#16440=ORIENTED_EDGE('',*,*,#12225,.T.);
#16441=ORIENTED_EDGE('',*,*,#12226,.F.);
#16442=ORIENTED_EDGE('',*,*,#12227,.F.);
#16443=ORIENTED_EDGE('',*,*,#12228,.T.);
#16444=ORIENTED_EDGE('',*,*,#12229,.T.);
#16445=ORIENTED_EDGE('',*,*,#12224,.F.);
#16446=ORIENTED_EDGE('',*,*,#12230,.F.);
#16447=ORIENTED_EDGE('',*,*,#12231,.T.);
#16448=ORIENTED_EDGE('',*,*,#12232,.T.);
#16449=ORIENTED_EDGE('',*,*,#12228,.F.);
#16450=ORIENTED_EDGE('',*,*,#12233,.F.);
#16451=ORIENTED_EDGE('',*,*,#12234,.T.);
#16452=ORIENTED_EDGE('',*,*,#12235,.T.);
#16453=ORIENTED_EDGE('',*,*,#12231,.F.);
#16454=ORIENTED_EDGE('',*,*,#12236,.F.);
#16455=ORIENTED_EDGE('',*,*,#12237,.T.);
#16456=ORIENTED_EDGE('',*,*,#12238,.T.);
#16457=ORIENTED_EDGE('',*,*,#12234,.F.);
#16458=ORIENTED_EDGE('',*,*,#12239,.F.);
#16459=ORIENTED_EDGE('',*,*,#12240,.T.);
#16460=ORIENTED_EDGE('',*,*,#12241,.T.);
#16461=ORIENTED_EDGE('',*,*,#12237,.F.);
#16462=ORIENTED_EDGE('',*,*,#12242,.F.);
#16463=ORIENTED_EDGE('',*,*,#12226,.T.);
#16464=ORIENTED_EDGE('',*,*,#12243,.T.);
#16465=ORIENTED_EDGE('',*,*,#12240,.F.);
#16466=ORIENTED_EDGE('',*,*,#12243,.F.);
#16467=ORIENTED_EDGE('',*,*,#12225,.F.);
#16468=ORIENTED_EDGE('',*,*,#12229,.F.);
#16469=ORIENTED_EDGE('',*,*,#12232,.F.);
#16470=ORIENTED_EDGE('',*,*,#12235,.F.);
#16471=ORIENTED_EDGE('',*,*,#12238,.F.);
#16472=ORIENTED_EDGE('',*,*,#12241,.F.);
#16473=ORIENTED_EDGE('',*,*,#12244,.T.);
#16474=ORIENTED_EDGE('',*,*,#12245,.T.);
#16475=ORIENTED_EDGE('',*,*,#12246,.T.);
#16476=ORIENTED_EDGE('',*,*,#12247,.T.);
#16477=ORIENTED_EDGE('',*,*,#12245,.F.);
#16478=ORIENTED_EDGE('',*,*,#12248,.F.);
#16479=ORIENTED_EDGE('',*,*,#12244,.F.);
#16480=ORIENTED_EDGE('',*,*,#12246,.F.);
#16481=ORIENTED_EDGE('',*,*,#12247,.F.);
#16482=ORIENTED_EDGE('',*,*,#12249,.T.);
#16483=ORIENTED_EDGE('',*,*,#12250,.F.);
#16484=ORIENTED_EDGE('',*,*,#12249,.F.);
#16485=ORIENTED_EDGE('',*,*,#12251,.T.);
#16486=ORIENTED_EDGE('',*,*,#12252,.T.);
#16487=ORIENTED_EDGE('',*,*,#12253,.T.);
#16488=ORIENTED_EDGE('',*,*,#12254,.T.);
#16489=ORIENTED_EDGE('',*,*,#12252,.F.);
#16490=ORIENTED_EDGE('',*,*,#12255,.F.);
#16491=ORIENTED_EDGE('',*,*,#12251,.F.);
#16492=ORIENTED_EDGE('',*,*,#12253,.F.);
#16493=ORIENTED_EDGE('',*,*,#12254,.F.);
#16494=ORIENTED_EDGE('',*,*,#12256,.T.);
#16495=ORIENTED_EDGE('',*,*,#12257,.F.);
#16496=ORIENTED_EDGE('',*,*,#12256,.F.);
#16497=ORIENTED_EDGE('',*,*,#12258,.T.);
#16498=ORIENTED_EDGE('',*,*,#12259,.T.);
#16499=ORIENTED_EDGE('',*,*,#12260,.T.);
#16500=ORIENTED_EDGE('',*,*,#12261,.T.);
#16501=ORIENTED_EDGE('',*,*,#12259,.F.);
#16502=ORIENTED_EDGE('',*,*,#12262,.F.);
#16503=ORIENTED_EDGE('',*,*,#12258,.F.);
#16504=ORIENTED_EDGE('',*,*,#12260,.F.);
#16505=ORIENTED_EDGE('',*,*,#12261,.F.);
#16506=ORIENTED_EDGE('',*,*,#12263,.T.);
#16507=ORIENTED_EDGE('',*,*,#12264,.F.);
#16508=ORIENTED_EDGE('',*,*,#12263,.F.);
#16509=ORIENTED_EDGE('',*,*,#12265,.T.);
#16510=ORIENTED_EDGE('',*,*,#12266,.T.);
#16511=ORIENTED_EDGE('',*,*,#12267,.T.);
#16512=ORIENTED_EDGE('',*,*,#12268,.T.);
#16513=ORIENTED_EDGE('',*,*,#12266,.F.);
#16514=ORIENTED_EDGE('',*,*,#12269,.F.);
#16515=ORIENTED_EDGE('',*,*,#12265,.F.);
#16516=ORIENTED_EDGE('',*,*,#12267,.F.);
#16517=ORIENTED_EDGE('',*,*,#12268,.F.);
#16518=ORIENTED_EDGE('',*,*,#12270,.T.);
#16519=ORIENTED_EDGE('',*,*,#12271,.F.);
#16520=ORIENTED_EDGE('',*,*,#12270,.F.);
#16521=ORIENTED_EDGE('',*,*,#12272,.T.);
#16522=ORIENTED_EDGE('',*,*,#12273,.T.);
#16523=ORIENTED_EDGE('',*,*,#12274,.T.);
#16524=ORIENTED_EDGE('',*,*,#12275,.T.);
#16525=ORIENTED_EDGE('',*,*,#12273,.F.);
#16526=ORIENTED_EDGE('',*,*,#12276,.F.);
#16527=ORIENTED_EDGE('',*,*,#12272,.F.);
#16528=ORIENTED_EDGE('',*,*,#12274,.F.);
#16529=ORIENTED_EDGE('',*,*,#12275,.F.);
#16530=ORIENTED_EDGE('',*,*,#12277,.T.);
#16531=ORIENTED_EDGE('',*,*,#12278,.F.);
#16532=ORIENTED_EDGE('',*,*,#12277,.F.);
#16533=ORIENTED_EDGE('',*,*,#12279,.T.);
#16534=ORIENTED_EDGE('',*,*,#12280,.T.);
#16535=ORIENTED_EDGE('',*,*,#12281,.T.);
#16536=ORIENTED_EDGE('',*,*,#12282,.T.);
#16537=ORIENTED_EDGE('',*,*,#12280,.F.);
#16538=ORIENTED_EDGE('',*,*,#12283,.F.);
#16539=ORIENTED_EDGE('',*,*,#12279,.F.);
#16540=ORIENTED_EDGE('',*,*,#12281,.F.);
#16541=ORIENTED_EDGE('',*,*,#12282,.F.);
#16542=ORIENTED_EDGE('',*,*,#12284,.T.);
#16543=ORIENTED_EDGE('',*,*,#12285,.F.);
#16544=ORIENTED_EDGE('',*,*,#12284,.F.);
#16545=ORIENTED_EDGE('',*,*,#12286,.F.);
#16546=ORIENTED_EDGE('',*,*,#12287,.F.);
#16547=ORIENTED_EDGE('',*,*,#12288,.F.);
#16548=ORIENTED_EDGE('',*,*,#12289,.T.);
#16549=ORIENTED_EDGE('',*,*,#12283,.T.);
#16550=ORIENTED_EDGE('',*,*,#12289,.F.);
#16551=ORIENTED_EDGE('',*,*,#12290,.T.);
#16552=ORIENTED_EDGE('',*,*,#12291,.T.);
#16553=ORIENTED_EDGE('',*,*,#12292,.T.);
#16554=ORIENTED_EDGE('',*,*,#12293,.T.);
#16555=ORIENTED_EDGE('',*,*,#12294,.T.);
#16556=ORIENTED_EDGE('',*,*,#12295,.T.);
#16557=ORIENTED_EDGE('',*,*,#12296,.T.);
#16558=ORIENTED_EDGE('',*,*,#12297,.T.);
#16559=ORIENTED_EDGE('',*,*,#12298,.T.);
#16560=ORIENTED_EDGE('',*,*,#12299,.T.);
#16561=ORIENTED_EDGE('',*,*,#12300,.T.);
#16562=ORIENTED_EDGE('',*,*,#12287,.T.);
#16563=ORIENTED_EDGE('',*,*,#12301,.T.);
#16564=ORIENTED_EDGE('',*,*,#12302,.T.);
#16565=ORIENTED_EDGE('',*,*,#12303,.T.);
#16566=ORIENTED_EDGE('',*,*,#12304,.T.);
#16567=ORIENTED_EDGE('',*,*,#12291,.F.);
#16568=ORIENTED_EDGE('',*,*,#12302,.F.);
#16569=ORIENTED_EDGE('',*,*,#12305,.F.);
#16570=ORIENTED_EDGE('',*,*,#12306,.T.);
#16571=ORIENTED_EDGE('',*,*,#12276,.T.);
#16572=ORIENTED_EDGE('',*,*,#12306,.F.);
#16573=ORIENTED_EDGE('',*,*,#12307,.F.);
#16574=ORIENTED_EDGE('',*,*,#12308,.F.);
#16575=ORIENTED_EDGE('',*,*,#12286,.T.);
#16576=ORIENTED_EDGE('',*,*,#12288,.T.);
#16577=ORIENTED_EDGE('',*,*,#12300,.F.);
#16578=ORIENTED_EDGE('',*,*,#12309,.T.);
#16579=ORIENTED_EDGE('',*,*,#12297,.F.);
#16580=ORIENTED_EDGE('',*,*,#12310,.T.);
#16581=ORIENTED_EDGE('',*,*,#12311,.T.);
#16582=ORIENTED_EDGE('',*,*,#12295,.F.);
#16583=ORIENTED_EDGE('',*,*,#12312,.T.);
#16584=ORIENTED_EDGE('',*,*,#12313,.T.);
#16585=ORIENTED_EDGE('',*,*,#12293,.F.);
#16586=ORIENTED_EDGE('',*,*,#12314,.T.);
#16587=ORIENTED_EDGE('',*,*,#12315,.T.);
#16588=ORIENTED_EDGE('',*,*,#12303,.F.);
#16589=ORIENTED_EDGE('',*,*,#12307,.T.);
#16590=ORIENTED_EDGE('',*,*,#12305,.T.);
#16591=ORIENTED_EDGE('',*,*,#12301,.F.);
#16592=ORIENTED_EDGE('',*,*,#12314,.F.);
#16593=ORIENTED_EDGE('',*,*,#12292,.F.);
#16594=ORIENTED_EDGE('',*,*,#12304,.F.);
#16595=ORIENTED_EDGE('',*,*,#12315,.F.);
#16596=ORIENTED_EDGE('',*,*,#12316,.T.);
#16597=ORIENTED_EDGE('',*,*,#12269,.T.);
#16598=ORIENTED_EDGE('',*,*,#12316,.F.);
#16599=ORIENTED_EDGE('',*,*,#12294,.F.);
#16600=ORIENTED_EDGE('',*,*,#12313,.F.);
#16601=ORIENTED_EDGE('',*,*,#12317,.T.);
#16602=ORIENTED_EDGE('',*,*,#12262,.T.);
#16603=ORIENTED_EDGE('',*,*,#12317,.F.);
#16604=ORIENTED_EDGE('',*,*,#12312,.F.);
#16605=ORIENTED_EDGE('',*,*,#12310,.F.);
#16606=ORIENTED_EDGE('',*,*,#12296,.F.);
#16607=ORIENTED_EDGE('',*,*,#12311,.F.);
#16608=ORIENTED_EDGE('',*,*,#12318,.T.);
#16609=ORIENTED_EDGE('',*,*,#12255,.T.);
#16610=ORIENTED_EDGE('',*,*,#12318,.F.);
#16611=ORIENTED_EDGE('',*,*,#12298,.F.);
#16612=ORIENTED_EDGE('',*,*,#12309,.F.);
#16613=ORIENTED_EDGE('',*,*,#12299,.F.);
#16614=ORIENTED_EDGE('',*,*,#12319,.T.);
#16615=ORIENTED_EDGE('',*,*,#12248,.T.);
#16616=ORIENTED_EDGE('',*,*,#12319,.F.);
#16617=ORIENTED_EDGE('',*,*,#12320,.T.);
#16618=ORIENTED_EDGE('',*,*,#12321,.T.);
#16619=ORIENTED_EDGE('',*,*,#12322,.T.);
#16620=ORIENTED_EDGE('',*,*,#12321,.F.);
#16621=ORIENTED_EDGE('',*,*,#12322,.F.);
#16622=ORIENTED_EDGE('',*,*,#12323,.T.);
#16623=ORIENTED_EDGE('',*,*,#12324,.F.);
#16624=ORIENTED_EDGE('',*,*,#12325,.F.);
#16625=ORIENTED_EDGE('',*,*,#12323,.F.);
#16626=ORIENTED_EDGE('',*,*,#12326,.F.);
#16627=ORIENTED_EDGE('',*,*,#12320,.F.);
#16628=ORIENTED_EDGE('',*,*,#12326,.T.);
#16629=ORIENTED_EDGE('',*,*,#12327,.T.);
#16630=ORIENTED_EDGE('',*,*,#12328,.T.);
#16631=ORIENTED_EDGE('',*,*,#12327,.F.);
#16632=ORIENTED_EDGE('',*,*,#12328,.F.);
#16633=ORIENTED_EDGE('',*,*,#12329,.T.);
#16634=ORIENTED_EDGE('',*,*,#12330,.F.);
#16635=ORIENTED_EDGE('',*,*,#12331,.F.);
#16636=ORIENTED_EDGE('',*,*,#12329,.F.);
#16637=ORIENTED_EDGE('',*,*,#12332,.T.);
#16638=ORIENTED_EDGE('',*,*,#12333,.T.);
#16639=ORIENTED_EDGE('',*,*,#12334,.T.);
#16640=ORIENTED_EDGE('',*,*,#12335,.T.);
#16641=ORIENTED_EDGE('',*,*,#12334,.F.);
#16642=ORIENTED_EDGE('',*,*,#12336,.T.);
#16643=ORIENTED_EDGE('',*,*,#12285,.T.);
#16644=ORIENTED_EDGE('',*,*,#12278,.T.);
#16645=ORIENTED_EDGE('',*,*,#12271,.T.);
#16646=ORIENTED_EDGE('',*,*,#12264,.T.);
#16647=ORIENTED_EDGE('',*,*,#12257,.T.);
#16648=ORIENTED_EDGE('',*,*,#12250,.T.);
#16649=ORIENTED_EDGE('',*,*,#12335,.F.);
#16650=ORIENTED_EDGE('',*,*,#12332,.F.);
#16651=ORIENTED_EDGE('',*,*,#12333,.F.);
#16652=ORIENTED_EDGE('',*,*,#12337,.T.);
#16653=ORIENTED_EDGE('',*,*,#12338,.F.);
#16654=ORIENTED_EDGE('',*,*,#12337,.F.);
#16655=ORIENTED_EDGE('',*,*,#12324,.T.);
#16656=ORIENTED_EDGE('',*,*,#12325,.T.);
#16657=ORIENTED_EDGE('',*,*,#12339,.T.);
#16658=ORIENTED_EDGE('',*,*,#12340,.T.);
#16659=ORIENTED_EDGE('',*,*,#12341,.T.);
#16660=ORIENTED_EDGE('',*,*,#12342,.T.);
#16661=ORIENTED_EDGE('',*,*,#12340,.F.);
#16662=ORIENTED_EDGE('',*,*,#12343,.T.);
#16663=ORIENTED_EDGE('',*,*,#12344,.T.);
#16664=ORIENTED_EDGE('',*,*,#12341,.F.);
#16665=ORIENTED_EDGE('',*,*,#12342,.F.);
#16666=ORIENTED_EDGE('',*,*,#12344,.F.);
#16667=ORIENTED_EDGE('',*,*,#12345,.F.);
#16668=ORIENTED_EDGE('',*,*,#12223,.T.);
#16669=ORIENTED_EDGE('',*,*,#12242,.T.);
#16670=ORIENTED_EDGE('',*,*,#12239,.T.);
#16671=ORIENTED_EDGE('',*,*,#12236,.T.);
#16672=ORIENTED_EDGE('',*,*,#12233,.T.);
#16673=ORIENTED_EDGE('',*,*,#12230,.T.);
#16674=ORIENTED_EDGE('',*,*,#12227,.T.);
#16675=ORIENTED_EDGE('',*,*,#12339,.F.);
#16676=ORIENTED_EDGE('',*,*,#12346,.T.);
#16677=ORIENTED_EDGE('',*,*,#12347,.T.);
#16678=ORIENTED_EDGE('',*,*,#12348,.T.);
#16679=ORIENTED_EDGE('',*,*,#12347,.F.);
#16680=ORIENTED_EDGE('',*,*,#12290,.F.);
#16681=ORIENTED_EDGE('',*,*,#12349,.T.);
#16682=ORIENTED_EDGE('',*,*,#12346,.F.);
#16683=ORIENTED_EDGE('',*,*,#12349,.F.);
#16684=ORIENTED_EDGE('',*,*,#12330,.T.);
#16685=ORIENTED_EDGE('',*,*,#12331,.T.);
#16686=ORIENTED_EDGE('',*,*,#12348,.F.);
#16687=ORIENTED_EDGE('',*,*,#12350,.T.);
#16688=ORIENTED_EDGE('',*,*,#12351,.T.);
#16689=ORIENTED_EDGE('',*,*,#12350,.F.);
#16690=ORIENTED_EDGE('',*,*,#12352,.F.);
#16691=ORIENTED_EDGE('',*,*,#12353,.T.);
#16692=ORIENTED_EDGE('',*,*,#12345,.T.);
#16693=ORIENTED_EDGE('',*,*,#12353,.F.);
#16694=ORIENTED_EDGE('',*,*,#12351,.F.);
#16695=ORIENTED_EDGE('',*,*,#12354,.T.);
#16696=ORIENTED_EDGE('',*,*,#12352,.T.);
#16697=ORIENTED_EDGE('',*,*,#12354,.F.);
#16698=ORIENTED_EDGE('',*,*,#12355,.F.);
#16699=ORIENTED_EDGE('',*,*,#12356,.T.);
#16700=ORIENTED_EDGE('',*,*,#12308,.T.);
#16701=ORIENTED_EDGE('',*,*,#12356,.F.);
#16702=ORIENTED_EDGE('',*,*,#12357,.F.);
#16703=ORIENTED_EDGE('',*,*,#12358,.T.);
#16704=ORIENTED_EDGE('',*,*,#12355,.T.);
#16705=ORIENTED_EDGE('',*,*,#12358,.F.);
#16706=ORIENTED_EDGE('',*,*,#12336,.F.);
#16707=ORIENTED_EDGE('',*,*,#12359,.T.);
#16708=ORIENTED_EDGE('',*,*,#12357,.T.);
#16709=ORIENTED_EDGE('',*,*,#12359,.F.);
#16710=ORIENTED_EDGE('',*,*,#12338,.T.);
#16711=ORIENTED_EDGE('',*,*,#12360,.F.);
#16712=ORIENTED_EDGE('',*,*,#12360,.T.);
#16713=ORIENTED_EDGE('',*,*,#12361,.T.);
#16714=ORIENTED_EDGE('',*,*,#12362,.F.);
#16715=ORIENTED_EDGE('',*,*,#12361,.F.);
#16716=ORIENTED_EDGE('',*,*,#12362,.T.);
#16717=ORIENTED_EDGE('',*,*,#12363,.F.);
#16718=ORIENTED_EDGE('',*,*,#12363,.T.);
#16719=ORIENTED_EDGE('',*,*,#12364,.T.);
#16720=ORIENTED_EDGE('',*,*,#12365,.F.);
#16721=ORIENTED_EDGE('',*,*,#12364,.F.);
#16722=ORIENTED_EDGE('',*,*,#12366,.F.);
#16723=ORIENTED_EDGE('',*,*,#12365,.T.);
#16724=ORIENTED_EDGE('',*,*,#12366,.T.);
#16725=ORIENTED_EDGE('',*,*,#12367,.T.);
#16726=ORIENTED_EDGE('',*,*,#12368,.F.);
#16727=ORIENTED_EDGE('',*,*,#12367,.F.);
#16728=ORIENTED_EDGE('',*,*,#12368,.T.);
#16729=ORIENTED_EDGE('',*,*,#12369,.F.);
#16730=ORIENTED_EDGE('',*,*,#12369,.T.);
#16731=ORIENTED_EDGE('',*,*,#12370,.T.);
#16732=ORIENTED_EDGE('',*,*,#12371,.F.);
#16733=ORIENTED_EDGE('',*,*,#12370,.F.);
#16734=ORIENTED_EDGE('',*,*,#12371,.T.);
#16735=ORIENTED_EDGE('',*,*,#12343,.F.);
#21367=CONICAL_SURFACE('',#23733,0.4625,0.785398163397455);
#21368=CONICAL_SURFACE('',#23741,0.4625,0.785398163397446);
#21369=CONICAL_SURFACE('',#23749,0.4625,0.785398163397446);
#21370=CONICAL_SURFACE('',#23757,0.4625,0.785398163397455);
#21371=CONICAL_SURFACE('',#23765,0.4625,0.785398163397446);
#21372=CONICAL_SURFACE('',#23773,0.4625,0.785398163397446);
#21373=CONICAL_SURFACE('',#23809,0.70285,0.785398163397448);
#21374=CONICAL_SURFACE('',#23815,1.25,0.785398163397448);
#21375=CONICAL_SURFACE('',#23818,4.325,0.785398163397448);
#21376=CONICAL_SURFACE('',#23826,2.05,0.785398163397451);
#21377=CONICAL_SURFACE('',#23839,4.1,0.963808662748489);
#21378=CONICAL_SURFACE('',#23841,3.15,0.785398163397451);
#21379=CONICAL_SURFACE('',#23844,6.95,0.785398163397447);
#21380=CONICAL_SURFACE('',#23848,6.975,0.463647609000805);
#21875=ADVANCED_FACE('',(#3045),#2020,.F.);
#21876=ADVANCED_FACE('',(#3046),#2021,.F.);
#21877=ADVANCED_FACE('',(#3047),#2022,.F.);
#21878=ADVANCED_FACE('',(#3048),#2023,.F.);
#21879=ADVANCED_FACE('',(#3049),#2504,.T.);
#21880=ADVANCED_FACE('',(#3050),#2024,.F.);
#21881=ADVANCED_FACE('',(#3051),#2505,.F.);
#21882=ADVANCED_FACE('',(#3052),#2025,.F.);
#21883=ADVANCED_FACE('',(#3053),#21367,.F.);
#21884=ADVANCED_FACE('',(#3054,#1670),#2026,.F.);
#21885=ADVANCED_FACE('',(#3055),#2506,.F.);
#21886=ADVANCED_FACE('',(#3056),#21368,.F.);
#21887=ADVANCED_FACE('',(#3057,#1671),#2027,.F.);
#21888=ADVANCED_FACE('',(#3058),#2507,.F.);
#21889=ADVANCED_FACE('',(#3059),#21369,.F.);
#21890=ADVANCED_FACE('',(#3060,#1672),#2028,.F.);
#21891=ADVANCED_FACE('',(#3061),#2508,.F.);
#21892=ADVANCED_FACE('',(#3062),#21370,.F.);
#21893=ADVANCED_FACE('',(#3063,#1673),#2029,.F.);
#21894=ADVANCED_FACE('',(#3064),#2509,.F.);
#21895=ADVANCED_FACE('',(#3065),#21371,.F.);
#21896=ADVANCED_FACE('',(#3066,#1674),#2030,.F.);
#21897=ADVANCED_FACE('',(#3067),#2510,.F.);
#21898=ADVANCED_FACE('',(#3068),#21372,.F.);
#21899=ADVANCED_FACE('',(#3069,#1675),#2031,.F.);
#21900=ADVANCED_FACE('',(#3070),#2511,.F.);
#21901=ADVANCED_FACE('',(#3071),#2512,.F.);
#21902=ADVANCED_FACE('',(#3072),#310,.F.);
#21903=ADVANCED_FACE('',(#3073),#2513,.F.);
#21904=ADVANCED_FACE('',(#3074,#1676),#2032,.T.);
#21905=ADVANCED_FACE('',(#3075),#2514,.F.);
#21906=ADVANCED_FACE('',(#3076),#2515,.F.);
#21907=ADVANCED_FACE('',(#3077),#2516,.F.);
#21908=ADVANCED_FACE('',(#3078),#2517,.F.);
#21909=ADVANCED_FACE('',(#3079),#21373,.F.);
#21910=ADVANCED_FACE('',(#3080),#2518,.F.);
#21911=ADVANCED_FACE('',(#3081,#1677),#2033,.T.);
#21912=ADVANCED_FACE('',(#3082),#21374,.T.);
#21913=ADVANCED_FACE('',(#3083),#2519,.T.);
#21914=ADVANCED_FACE('',(#3084),#21375,.F.);
#21915=ADVANCED_FACE('',(#3085,#1678,#1679,#1680,#1681,#1682,#1683,#1684),
#2034,.T.);
#21916=ADVANCED_FACE('',(#3086,#1685),#2520,.F.);
#21917=ADVANCED_FACE('',(#3087),#21376,.F.);
#21918=ADVANCED_FACE('',(#3088),#2521,.F.);
#21919=ADVANCED_FACE('',(#3089,#1686,#1687),#2035,.T.);
#21920=ADVANCED_FACE('',(#3090),#311,.T.);
#21921=ADVANCED_FACE('',(#3091,#1688),#2522,.T.);
#21922=ADVANCED_FACE('',(#3092),#21377,.T.);
#21923=ADVANCED_FACE('',(#3093),#21378,.T.);
#21924=ADVANCED_FACE('',(#3094),#2523,.T.);
#21925=ADVANCED_FACE('',(#3095),#21379,.T.);
#21926=ADVANCED_FACE('',(#3096),#2524,.T.);
#21927=ADVANCED_FACE('',(#3097),#21380,.T.);
#21928=ADVANCED_FACE('',(#3098,#1689),#2036,.T.);
#21929=ADVANCED_FACE('',(#3099),#2525,.F.);
#21930=ADVANCED_FACE('',(#3100,#1690),#2037,.T.);
#21931=ADVANCED_FACE('',(#3101),#2526,.F.);
#21932=ADVANCED_FACE('',(#3102,#1691),#2038,.T.);
#21933=ADVANCED_FACE('',(#3103),#2527,.F.);
#21934=ADVANCED_FACE('',(#3104,#1692),#2039,.T.);
#21935=ADVANCED_FACE('',(#3105),#2528,.F.);
#21936=ADVANCED_FACE('',(#3106,#1693),#2040,.T.);
#22814=CLOSED_SHELL('',(#21875,#21876,#21877,#21878,#21879,#21880,#21881,
#21882,#21883,#21884,#21885,#21886,#21887,#21888,#21889,#21890,#21891,#21892,
#21893,#21894,#21895,#21896,#21897,#21898,#21899,#21900,#21901,#21902,#21903,
#21904,#21905,#21906,#21907,#21908,#21909,#21910,#21911,#21912,#21913,#21914,
#21915,#21916,#21917,#21918,#21919,#21920,#21921,#21922,#21923,#21924,#21925,
#21926,#21927,#21928,#21929,#21930,#21931,#21932,#21933,#21934,#21935,#21936));
#23720=AXIS2_PLACEMENT_3D('',#42303,#26895,#26896);
#23721=AXIS2_PLACEMENT_3D('',#42304,#26897,#26898);
#23722=AXIS2_PLACEMENT_3D('',#42313,#26903,#26904);
#23723=AXIS2_PLACEMENT_3D('',#42319,#26908,#26909);
#23724=AXIS2_PLACEMENT_3D('',#42325,#26913,#26914);
#23725=AXIS2_PLACEMENT_3D('',#42331,#26918,#26919);
#23726=AXIS2_PLACEMENT_3D('',#42333,#26920,#26921);
#23727=AXIS2_PLACEMENT_3D('',#42336,#26923,#26924);
#23728=AXIS2_PLACEMENT_3D('',#42337,#26925,#26926);
#23729=AXIS2_PLACEMENT_3D('',#42343,#26930,#26931);
#23730=AXIS2_PLACEMENT_3D('',#42344,#26932,#26933);
#23731=AXIS2_PLACEMENT_3D('',#42345,#26934,#26935);
#23732=AXIS2_PLACEMENT_3D('',#42346,#26936,#26937);
#23733=AXIS2_PLACEMENT_3D('',#42347,#26938,#26939);
#23734=AXIS2_PLACEMENT_3D('',#42349,#26940,#26941);
#23735=AXIS2_PLACEMENT_3D('',#42353,#26943,#26944);
#23736=AXIS2_PLACEMENT_3D('',#42354,#26945,#26946);
#23737=AXIS2_PLACEMENT_3D('',#42355,#26947,#26948);
#23738=AXIS2_PLACEMENT_3D('',#42357,#26949,#26950);
#23739=AXIS2_PLACEMENT_3D('',#42358,#26951,#26952);
#23740=AXIS2_PLACEMENT_3D('',#42361,#26954,#26955);
#23741=AXIS2_PLACEMENT_3D('',#42362,#26956,#26957);
#23742=AXIS2_PLACEMENT_3D('',#42364,#26958,#26959);
#23743=AXIS2_PLACEMENT_3D('',#42368,#26961,#26962);
#23744=AXIS2_PLACEMENT_3D('',#42369,#26963,#26964);
#23745=AXIS2_PLACEMENT_3D('',#42370,#26965,#26966);
#23746=AXIS2_PLACEMENT_3D('',#42372,#26967,#26968);
#23747=AXIS2_PLACEMENT_3D('',#42373,#26969,#26970);
#23748=AXIS2_PLACEMENT_3D('',#42376,#26972,#26973);
#23749=AXIS2_PLACEMENT_3D('',#42377,#26974,#26975);
#23750=AXIS2_PLACEMENT_3D('',#42379,#26976,#26977);
#23751=AXIS2_PLACEMENT_3D('',#42383,#26979,#26980);
#23752=AXIS2_PLACEMENT_3D('',#42384,#26981,#26982);
#23753=AXIS2_PLACEMENT_3D('',#42385,#26983,#26984);
#23754=AXIS2_PLACEMENT_3D('',#42387,#26985,#26986);
#23755=AXIS2_PLACEMENT_3D('',#42388,#26987,#26988);
#23756=AXIS2_PLACEMENT_3D('',#42391,#26990,#26991);
#23757=AXIS2_PLACEMENT_3D('',#42392,#26992,#26993);
#23758=AXIS2_PLACEMENT_3D('',#42394,#26994,#26995);
#23759=AXIS2_PLACEMENT_3D('',#42398,#26997,#26998);
#23760=AXIS2_PLACEMENT_3D('',#42399,#26999,#27000);
#23761=AXIS2_PLACEMENT_3D('',#42400,#27001,#27002);
#23762=AXIS2_PLACEMENT_3D('',#42402,#27003,#27004);
#23763=AXIS2_PLACEMENT_3D('',#42403,#27005,#27006);
#23764=AXIS2_PLACEMENT_3D('',#42406,#27008,#27009);
#23765=AXIS2_PLACEMENT_3D('',#42407,#27010,#27011);
#23766=AXIS2_PLACEMENT_3D('',#42409,#27012,#27013);
#23767=AXIS2_PLACEMENT_3D('',#42413,#27015,#27016);
#23768=AXIS2_PLACEMENT_3D('',#42414,#27017,#27018);
#23769=AXIS2_PLACEMENT_3D('',#42415,#27019,#27020);
#23770=AXIS2_PLACEMENT_3D('',#42417,#27021,#27022);
#23771=AXIS2_PLACEMENT_3D('',#42418,#27023,#27024);
#23772=AXIS2_PLACEMENT_3D('',#42421,#27026,#27027);
#23773=AXIS2_PLACEMENT_3D('',#42422,#27028,#27029);
#23774=AXIS2_PLACEMENT_3D('',#42424,#27030,#27031);
#23775=AXIS2_PLACEMENT_3D('',#42428,#27033,#27034);
#23776=AXIS2_PLACEMENT_3D('',#42429,#27035,#27036);
#23777=AXIS2_PLACEMENT_3D('',#42430,#27037,#27038);
#23778=AXIS2_PLACEMENT_3D('',#42432,#27039,#27040);
#23779=AXIS2_PLACEMENT_3D('',#42433,#27041,#27042);
#23780=AXIS2_PLACEMENT_3D('',#42436,#27044,#27045);
#23781=AXIS2_PLACEMENT_3D('',#42437,#27046,#27047);
#23782=AXIS2_PLACEMENT_3D('',#42440,#27048,#27049);
#23783=AXIS2_PLACEMENT_3D('',#42458,#27050,#27051);
#23784=AXIS2_PLACEMENT_3D('',#42460,#27053,#27054);
#23785=AXIS2_PLACEMENT_3D('',#42462,#27055,#27056);
#23786=AXIS2_PLACEMENT_3D('',#42464,#27057,#27058);
#23787=AXIS2_PLACEMENT_3D('',#42477,#27059,#27060);
#23788=AXIS2_PLACEMENT_3D('',#42496,#27061,#27062);
#23789=AXIS2_PLACEMENT_3D('',#42515,#27063,#27064);
#23790=AXIS2_PLACEMENT_3D('',#42538,#27065,#27066);
#23791=AXIS2_PLACEMENT_3D('',#42540,#27067,#27068);
#23792=AXIS2_PLACEMENT_3D('',#42559,#27069,#27070);
#23793=AXIS2_PLACEMENT_3D('',#42570,#27071,#27072);
#23794=AXIS2_PLACEMENT_3D('',#42572,#27073,#27074);
#23795=AXIS2_PLACEMENT_3D('',#42574,#27076,#27077);
#23796=AXIS2_PLACEMENT_3D('',#42575,#27078,#27079);
#23797=AXIS2_PLACEMENT_3D('',#42577,#27080,#27081);
#23798=AXIS2_PLACEMENT_3D('',#42578,#27082,#27083);
#23799=AXIS2_PLACEMENT_3D('',#42580,#27084,#27085);
#23800=AXIS2_PLACEMENT_3D('',#42581,#27086,#27087);
#23801=AXIS2_PLACEMENT_3D('',#42583,#27088,#27089);
#23802=AXIS2_PLACEMENT_3D('',#42584,#27090,#27091);
#23803=AXIS2_PLACEMENT_3D('',#42586,#27092,#27093);
#23804=AXIS2_PLACEMENT_3D('',#42587,#27094,#27095);
#23805=AXIS2_PLACEMENT_3D('',#42588,#27096,#27097);
#23806=AXIS2_PLACEMENT_3D('',#42590,#27099,#27100);
#23807=AXIS2_PLACEMENT_3D('',#42592,#27102,#27103);
#23808=AXIS2_PLACEMENT_3D('',#42594,#27105,#27106);
#23809=AXIS2_PLACEMENT_3D('',#42596,#27108,#27109);
#23810=AXIS2_PLACEMENT_3D('',#42598,#27110,#27111);
#23811=AXIS2_PLACEMENT_3D('',#42601,#27113,#27114);
#23812=AXIS2_PLACEMENT_3D('',#42602,#27115,#27116);
#23813=AXIS2_PLACEMENT_3D('',#42642,#27118,#27119);
#23814=AXIS2_PLACEMENT_3D('',#42644,#27120,#27121);
#23815=AXIS2_PLACEMENT_3D('',#42645,#27122,#27123);
#23816=AXIS2_PLACEMENT_3D('',#42648,#27125,#27126);
#23817=AXIS2_PLACEMENT_3D('',#42649,#27127,#27128);
#23818=AXIS2_PLACEMENT_3D('',#42689,#27130,#27131);
#23819=AXIS2_PLACEMENT_3D('',#42692,#27132,#27133);
#23820=AXIS2_PLACEMENT_3D('',#42693,#27134,#27135);
#23821=AXIS2_PLACEMENT_3D('',#42696,#27137,#27138);
#23822=AXIS2_PLACEMENT_3D('',#42697,#27139,#27140);
#23823=AXIS2_PLACEMENT_3D('',#42699,#27141,#27142);
#23824=AXIS2_PLACEMENT_3D('',#42700,#27143,#27144);
#23825=AXIS2_PLACEMENT_3D('',#42703,#27146,#27147);
#23826=AXIS2_PLACEMENT_3D('',#42704,#27148,#27149);
#23827=AXIS2_PLACEMENT_3D('',#42706,#27150,#27151);
#23828=AXIS2_PLACEMENT_3D('',#42710,#27153,#27154);
#23829=AXIS2_PLACEMENT_3D('',#42711,#27155,#27156);
#23830=AXIS2_PLACEMENT_3D('',#42712,#27157,#27158);
#23831=AXIS2_PLACEMENT_3D('',#42714,#27159,#27160);
#23832=AXIS2_PLACEMENT_3D('',#42716,#27162,#27163);
#23833=AXIS2_PLACEMENT_3D('',#42718,#27164,#27165);
#23834=AXIS2_PLACEMENT_3D('',#42719,#27166,#27167);
#23835=AXIS2_PLACEMENT_3D('',#42721,#27168,#27169);
#23836=AXIS2_PLACEMENT_3D('',#42723,#27170,#27171);
#23837=AXIS2_PLACEMENT_3D('',#42724,#27172,#27173);
#23838=AXIS2_PLACEMENT_3D('',#42725,#27174,#27175);
#23839=AXIS2_PLACEMENT_3D('',#42727,#27177,#27178);
#23840=AXIS2_PLACEMENT_3D('',#42730,#27180,#27181);
#23841=AXIS2_PLACEMENT_3D('',#42731,#27182,#27183);
#23842=AXIS2_PLACEMENT_3D('',#42733,#27184,#27185);
#23843=AXIS2_PLACEMENT_3D('',#42735,#27187,#27188);
#23844=AXIS2_PLACEMENT_3D('',#42737,#27190,#27191);
#23845=AXIS2_PLACEMENT_3D('',#42739,#27192,#27193);
#23846=AXIS2_PLACEMENT_3D('',#42741,#27195,#27196);
#23847=AXIS2_PLACEMENT_3D('',#42743,#27197,#27198);
#23848=AXIS2_PLACEMENT_3D('',#42745,#27200,#27201);
#23849=AXIS2_PLACEMENT_3D('',#42747,#27203,#27204);
#23850=AXIS2_PLACEMENT_3D('',#42749,#27205,#27206);
#23851=AXIS2_PLACEMENT_3D('',#42750,#27207,#27208);
#23852=AXIS2_PLACEMENT_3D('',#42753,#27210,#27211);
#23853=AXIS2_PLACEMENT_3D('',#42754,#27212,#27213);
#23854=AXIS2_PLACEMENT_3D('',#42756,#27214,#27215);
#23855=AXIS2_PLACEMENT_3D('',#42757,#27216,#27217);
#23856=AXIS2_PLACEMENT_3D('',#42760,#27219,#27220);
#23857=AXIS2_PLACEMENT_3D('',#42761,#27221,#27222);
#23858=AXIS2_PLACEMENT_3D('',#42763,#27223,#27224);
#23859=AXIS2_PLACEMENT_3D('',#42764,#27225,#27226);
#23860=AXIS2_PLACEMENT_3D('',#42767,#27228,#27229);
#23861=AXIS2_PLACEMENT_3D('',#42768,#27230,#27231);
#23862=AXIS2_PLACEMENT_3D('',#42770,#27232,#27233);
#23863=AXIS2_PLACEMENT_3D('',#42771,#27234,#27235);
#23864=AXIS2_PLACEMENT_3D('',#42774,#27237,#27238);
#23865=AXIS2_PLACEMENT_3D('',#42775,#27239,#27240);
#26895=DIRECTION('axis',(0.,0.,1.));
#26896=DIRECTION('refdir',(1.,0.,0.));
#26897=DIRECTION('center_axis',(-0.707106781186548,0.707106781186548,0.));
#26898=DIRECTION('ref_axis',(-0.707106781186548,-0.707106781186548,0.));
#26899=DIRECTION('',(-0.707106781186548,-0.707106781186548,0.));
#26900=DIRECTION('',(0.,0.,1.));
#26901=DIRECTION('',(-0.707106781186548,-0.707106781186548,0.));
#26902=DIRECTION('',(0.,0.,1.));
#26903=DIRECTION('center_axis',(0.977766079918218,0.20969857644095,0.));
#26904=DIRECTION('ref_axis',(-0.20969857644095,0.977766079918218,0.));
#26905=DIRECTION('',(-0.20969857644095,0.977766079918218,0.));
#26906=DIRECTION('',(0.,0.,1.));
#26907=DIRECTION('',(-0.20969857644095,0.977766079918218,0.));
#26908=DIRECTION('center_axis',(-0.407020185134245,-0.913419163852656,0.));
#26909=DIRECTION('ref_axis',(0.913419163852656,-0.407020185134245,0.));
#26910=DIRECTION('',(0.913419163852656,-0.407020185134245,0.));
#26911=DIRECTION('',(0.,0.,1.));
#26912=DIRECTION('',(0.913419163852656,-0.407020185134245,0.));
#26913=DIRECTION('center_axis',(-0.707106781186548,0.707106781186548,0.));
#26914=DIRECTION('ref_axis',(-0.707106781186548,-0.707106781186548,0.));
#26915=DIRECTION('',(-0.707106781186548,-0.707106781186548,0.));
#26916=DIRECTION('',(0.,0.,1.));
#26917=DIRECTION('',(-0.707106781186548,-0.707106781186548,0.));
#26918=DIRECTION('center_axis',(0.,0.,1.));
#26919=DIRECTION('ref_axis',(0.707106781186547,0.707106781186548,0.));
#26920=DIRECTION('center_axis',(0.,0.,-1.));
#26921=DIRECTION('ref_axis',(0.707106781186547,0.707106781186548,0.));
#26922=DIRECTION('',(0.,0.,1.));
#26923=DIRECTION('center_axis',(0.,0.,-1.));
#26924=DIRECTION('ref_axis',(0.707106781186547,0.707106781186548,0.));
#26925=DIRECTION('center_axis',(-0.707106781186547,-0.707106781186548,0.));
#26926=DIRECTION('ref_axis',(0.707106781186548,-0.707106781186547,0.));
#26927=DIRECTION('',(0.707106781186548,-0.707106781186547,0.));
#26928=DIRECTION('',(0.,0.,1.));
#26929=DIRECTION('',(0.707106781186548,-0.707106781186547,0.));
#26930=DIRECTION('center_axis',(0.,0.,1.));
#26931=DIRECTION('ref_axis',(0.707106781186548,0.707106781186547,0.));
#26932=DIRECTION('center_axis',(0.,0.,1.));
#26933=DIRECTION('ref_axis',(0.707106781186548,0.707106781186547,0.));
#26934=DIRECTION('center_axis',(0.,0.,1.));
#26935=DIRECTION('ref_axis',(0.707106781186548,0.707106781186547,0.));
#26936=DIRECTION('center_axis',(0.,0.,1.));
#26937=DIRECTION('ref_axis',(1.,0.,0.));
#26938=DIRECTION('center_axis',(0.,0.,-1.));
#26939=DIRECTION('ref_axis',(-1.,0.,0.));
#26940=DIRECTION('center_axis',(0.,0.,-1.));
#26941=DIRECTION('ref_axis',(-1.,0.,0.));
#26942=DIRECTION('',(-0.707106781186552,8.65956056235499E-17,0.707106781186543));
#26943=DIRECTION('center_axis',(0.,0.,1.));
#26944=DIRECTION('ref_axis',(-1.,0.,0.));
#26945=DIRECTION('center_axis',(0.,0.,1.));
#26946=DIRECTION('ref_axis',(-1.,0.,0.));
#26947=DIRECTION('center_axis',(0.,0.,1.));
#26948=DIRECTION('ref_axis',(1.,0.,0.));
#26949=DIRECTION('center_axis',(0.,0.,1.));
#26950=DIRECTION('ref_axis',(1.,0.,0.));
#26951=DIRECTION('center_axis',(0.,0.,1.));
#26952=DIRECTION('ref_axis',(1.,0.,0.));
#26953=DIRECTION('',(0.,0.,1.));
#26954=DIRECTION('center_axis',(0.,0.,-1.));
#26955=DIRECTION('ref_axis',(1.,0.,0.));
#26956=DIRECTION('center_axis',(0.,0.,-1.));
#26957=DIRECTION('ref_axis',(-1.,0.,0.));
#26958=DIRECTION('center_axis',(0.,0.,-1.));
#26959=DIRECTION('ref_axis',(-1.,0.,0.));
#26960=DIRECTION('',(-0.707106781186546,8.65956056235491E-17,0.707106781186549));
#26961=DIRECTION('center_axis',(0.,0.,1.));
#26962=DIRECTION('ref_axis',(-1.,0.,0.));
#26963=DIRECTION('center_axis',(0.,0.,1.));
#26964=DIRECTION('ref_axis',(-1.,0.,0.));
#26965=DIRECTION('center_axis',(0.,0.,1.));
#26966=DIRECTION('ref_axis',(1.,0.,0.));
#26967=DIRECTION('center_axis',(0.,0.,1.));
#26968=DIRECTION('ref_axis',(1.,0.,0.));
#26969=DIRECTION('center_axis',(0.,0.,1.));
#26970=DIRECTION('ref_axis',(1.,0.,0.));
#26971=DIRECTION('',(0.,0.,1.));
#26972=DIRECTION('center_axis',(0.,0.,-1.));
#26973=DIRECTION('ref_axis',(1.,0.,0.));
#26974=DIRECTION('center_axis',(0.,0.,-1.));
#26975=DIRECTION('ref_axis',(-1.,0.,0.));
#26976=DIRECTION('center_axis',(0.,0.,-1.));
#26977=DIRECTION('ref_axis',(-1.,0.,0.));
#26978=DIRECTION('',(-0.707106781186546,8.65956056235491E-17,0.707106781186549));
#26979=DIRECTION('center_axis',(0.,0.,1.));
#26980=DIRECTION('ref_axis',(-1.,0.,0.));
#26981=DIRECTION('center_axis',(0.,0.,1.));
#26982=DIRECTION('ref_axis',(-1.,0.,0.));
#26983=DIRECTION('center_axis',(0.,0.,1.));
#26984=DIRECTION('ref_axis',(1.,0.,0.));
#26985=DIRECTION('center_axis',(0.,0.,1.));
#26986=DIRECTION('ref_axis',(1.,0.,0.));
#26987=DIRECTION('center_axis',(0.,0.,1.));
#26988=DIRECTION('ref_axis',(1.,0.,0.));
#26989=DIRECTION('',(0.,0.,1.));
#26990=DIRECTION('center_axis',(0.,0.,-1.));
#26991=DIRECTION('ref_axis',(1.,0.,0.));
#26992=DIRECTION('center_axis',(0.,0.,-1.));
#26993=DIRECTION('ref_axis',(-1.,0.,0.));
#26994=DIRECTION('center_axis',(0.,0.,-1.));
#26995=DIRECTION('ref_axis',(-1.,0.,0.));
#26996=DIRECTION('',(-0.707106781186552,8.65956056235499E-17,0.707106781186543));
#26997=DIRECTION('center_axis',(0.,0.,1.));
#26998=DIRECTION('ref_axis',(-1.,0.,0.));
#26999=DIRECTION('center_axis',(0.,0.,1.));
#27000=DIRECTION('ref_axis',(-1.,0.,0.));
#27001=DIRECTION('center_axis',(0.,0.,1.));
#27002=DIRECTION('ref_axis',(1.,0.,0.));
#27003=DIRECTION('center_axis',(0.,0.,1.));
#27004=DIRECTION('ref_axis',(1.,0.,0.));
#27005=DIRECTION('center_axis',(0.,0.,1.));
#27006=DIRECTION('ref_axis',(1.,0.,0.));
#27007=DIRECTION('',(0.,0.,1.));
#27008=DIRECTION('center_axis',(0.,0.,-1.));
#27009=DIRECTION('ref_axis',(1.,0.,0.));
#27010=DIRECTION('center_axis',(0.,0.,-1.));
#27011=DIRECTION('ref_axis',(-1.,0.,0.));
#27012=DIRECTION('center_axis',(0.,0.,-1.));
#27013=DIRECTION('ref_axis',(-1.,0.,0.));
#27014=DIRECTION('',(-0.707106781186546,8.65956056235491E-17,0.707106781186549));
#27015=DIRECTION('center_axis',(0.,0.,1.));
#27016=DIRECTION('ref_axis',(-1.,0.,0.));
#27017=DIRECTION('center_axis',(0.,0.,1.));
#27018=DIRECTION('ref_axis',(-1.,0.,0.));
#27019=DIRECTION('center_axis',(0.,0.,1.));
#27020=DIRECTION('ref_axis',(1.,0.,0.));
#27021=DIRECTION('center_axis',(0.,0.,1.));
#27022=DIRECTION('ref_axis',(1.,0.,0.));
#27023=DIRECTION('center_axis',(0.,0.,1.));
#27024=DIRECTION('ref_axis',(1.,0.,0.));
#27025=DIRECTION('',(0.,0.,1.));
#27026=DIRECTION('center_axis',(0.,0.,-1.));
#27027=DIRECTION('ref_axis',(1.,0.,0.));
#27028=DIRECTION('center_axis',(0.,0.,-1.));
#27029=DIRECTION('ref_axis',(-1.,0.,0.));
#27030=DIRECTION('center_axis',(0.,0.,-1.));
#27031=DIRECTION('ref_axis',(-1.,0.,0.));
#27032=DIRECTION('',(-0.707106781186546,8.65956056235491E-17,0.707106781186549));
#27033=DIRECTION('center_axis',(0.,0.,1.));
#27034=DIRECTION('ref_axis',(-1.,0.,0.));
#27035=DIRECTION('center_axis',(0.,0.,1.));
#27036=DIRECTION('ref_axis',(-1.,0.,0.));
#27037=DIRECTION('center_axis',(0.,0.,1.));
#27038=DIRECTION('ref_axis',(1.,0.,0.));
#27039=DIRECTION('center_axis',(0.,0.,1.));
#27040=DIRECTION('ref_axis',(1.,0.,0.));
#27041=DIRECTION('center_axis',(0.,0.,1.));
#27042=DIRECTION('ref_axis',(1.,0.,0.));
#27043=DIRECTION('',(0.,0.,1.));
#27044=DIRECTION('center_axis',(0.,0.,-1.));
#27045=DIRECTION('ref_axis',(1.,0.,0.));
#27046=DIRECTION('center_axis',(0.,0.,1.));
#27047=DIRECTION('ref_axis',(1.,0.,0.));
#27048=DIRECTION('center_axis',(0.,0.,1.));
#27049=DIRECTION('ref_axis',(1.,0.,0.));
#27050=DIRECTION('center_axis',(0.,0.,1.));
#27051=DIRECTION('ref_axis',(1.,0.,0.));
#27052=DIRECTION('',(0.,0.,1.));
#27053=DIRECTION('center_axis',(0.,0.,1.));
#27054=DIRECTION('ref_axis',(1.,0.,0.));
#27055=DIRECTION('center_axis',(0.,0.,1.));
#27056=DIRECTION('ref_axis',(-1.,1.22464679914735E-16,0.));
#27057=DIRECTION('center_axis',(1.22464679914735E-16,-1.,0.));
#27058=DIRECTION('ref_axis',(-1.,-1.22464679914735E-16,0.));
#27059=DIRECTION('center_axis',(0.,0.,-1.));
#27060=DIRECTION('ref_axis',(-1.,1.22464679914735E-16,0.));
#27061=DIRECTION('center_axis',(0.,0.,-1.));
#27062=DIRECTION('ref_axis',(-1.,1.22464679914735E-16,0.));
#27063=DIRECTION('center_axis',(0.,0.,-1.));
#27064=DIRECTION('ref_axis',(-1.,1.22464679914735E-16,0.));
#27065=DIRECTION('center_axis',(0.,0.,-1.));
#27066=DIRECTION('ref_axis',(-1.,1.22464679914735E-16,0.));
#27067=DIRECTION('center_axis',(0.,0.,-1.));
#27068=DIRECTION('ref_axis',(-1.,1.22464679914735E-16,0.));
#27069=DIRECTION('center_axis',(0.,0.,-1.));
#27070=DIRECTION('ref_axis',(-1.,1.22464679914735E-16,0.));
#27071=DIRECTION('center_axis',(0.,0.,1.));
#27072=DIRECTION('ref_axis',(1.,0.,0.));
#27073=DIRECTION('center_axis',(0.,0.,1.));
#27074=DIRECTION('ref_axis',(1.,0.,0.));
#27075=DIRECTION('',(0.,0.,1.));
#27076=DIRECTION('center_axis',(0.,0.,1.));
#27077=DIRECTION('ref_axis',(1.,0.,0.));
#27078=DIRECTION('center_axis',(0.,0.,-1.));
#27079=DIRECTION('ref_axis',(-1.,0.,0.));
#27080=DIRECTION('center_axis',(0.,0.,1.));
#27081=DIRECTION('ref_axis',(1.,0.,0.));
#27082=DIRECTION('center_axis',(0.,0.,1.));
#27083=DIRECTION('ref_axis',(1.,0.,0.));
#27084=DIRECTION('center_axis',(0.,0.,1.));
#27085=DIRECTION('ref_axis',(1.,0.,0.));
#27086=DIRECTION('center_axis',(0.,0.,1.));
#27087=DIRECTION('ref_axis',(1.,0.,0.));
#27088=DIRECTION('center_axis',(0.,0.,1.));
#27089=DIRECTION('ref_axis',(1.,0.,0.));
#27090=DIRECTION('center_axis',(0.,0.,1.));
#27091=DIRECTION('ref_axis',(1.,0.,0.));
#27092=DIRECTION('center_axis',(0.,0.,1.));
#27093=DIRECTION('ref_axis',(1.,0.,0.));
#27094=DIRECTION('center_axis',(0.,0.,1.));
#27095=DIRECTION('ref_axis',(1.,0.,0.));
#27096=DIRECTION('center_axis',(0.,0.,1.));
#27097=DIRECTION('ref_axis',(1.,0.,0.));
#27098=DIRECTION('',(0.,0.,1.));
#27099=DIRECTION('center_axis',(0.,0.,1.));
#27100=DIRECTION('ref_axis',(1.,0.,0.));
#27101=DIRECTION('',(0.,0.,1.));
#27102=DIRECTION('center_axis',(0.,0.,1.));
#27103=DIRECTION('ref_axis',(1.,0.,0.));
#27104=DIRECTION('',(0.,0.,1.));
#27105=DIRECTION('center_axis',(0.,0.,1.));
#27106=DIRECTION('ref_axis',(1.,0.,0.));
#27107=DIRECTION('',(0.,0.,1.));
#27108=DIRECTION('center_axis',(1.,0.,0.));
#27109=DIRECTION('ref_axis',(0.,0.,1.));
#27110=DIRECTION('center_axis',(1.,0.,0.));
#27111=DIRECTION('ref_axis',(0.,0.,1.));
#27112=DIRECTION('',(-0.707106781186547,-8.65956056235493E-17,0.707106781186547));
#27113=DIRECTION('center_axis',(-1.,0.,0.));
#27114=DIRECTION('ref_axis',(0.,0.,1.));
#27115=DIRECTION('center_axis',(-1.,0.,0.));
#27116=DIRECTION('ref_axis',(0.,0.,1.));
#27117=DIRECTION('',(-1.,0.,0.));
#27118=DIRECTION('center_axis',(1.,0.,0.));
#27119=DIRECTION('ref_axis',(0.,0.,-1.));
#27120=DIRECTION('center_axis',(-1.,0.,0.));
#27121=DIRECTION('ref_axis',(0.,0.,-1.));
#27122=DIRECTION('center_axis',(-1.,0.,0.));
#27123=DIRECTION('ref_axis',(0.,0.,-1.));
#27124=DIRECTION('',(-0.707106781186548,-8.65956056235493E-17,0.707106781186548));
#27125=DIRECTION('center_axis',(1.,0.,0.));
#27126=DIRECTION('ref_axis',(0.,0.,-1.));
#27127=DIRECTION('center_axis',(1.,0.,0.));
#27128=DIRECTION('ref_axis',(0.,0.,-1.));
#27129=DIRECTION('',(-1.,0.,0.));
#27130=DIRECTION('center_axis',(0.,0.,1.));
#27131=DIRECTION('ref_axis',(-1.,0.,0.));
#27132=DIRECTION('center_axis',(0.,0.,-1.));
#27133=DIRECTION('ref_axis',(-1.,0.,0.));
#27134=DIRECTION('center_axis',(0.,0.,-1.));
#27135=DIRECTION('ref_axis',(-1.,0.,0.));
#27136=DIRECTION('',(0.707106781186547,-8.65956056235493E-17,0.707106781186547));
#27137=DIRECTION('center_axis',(0.,0.,1.));
#27138=DIRECTION('ref_axis',(-1.,0.,0.));
#27139=DIRECTION('center_axis',(0.,0.,1.));
#27140=DIRECTION('ref_axis',(1.,0.,0.));
#27141=DIRECTION('center_axis',(0.,0.,1.));
#27142=DIRECTION('ref_axis',(1.,0.,0.));
#27143=DIRECTION('center_axis',(0.,0.,1.));
#27144=DIRECTION('ref_axis',(1.,0.,0.));
#27145=DIRECTION('',(0.,0.,-1.));
#27146=DIRECTION('center_axis',(0.,0.,1.));
#27147=DIRECTION('ref_axis',(1.,0.,0.));
#27148=DIRECTION('center_axis',(0.,0.,-1.));
#27149=DIRECTION('ref_axis',(-1.,0.,0.));
#27150=DIRECTION('center_axis',(0.,0.,-1.));
#27151=DIRECTION('ref_axis',(-1.,0.,0.));
#27152=DIRECTION('',(-0.707106781186549,8.65956056235495E-17,0.707106781186546));
#27153=DIRECTION('center_axis',(0.,0.,1.));
#27154=DIRECTION('ref_axis',(-1.,0.,0.));
#27155=DIRECTION('center_axis',(0.,0.,1.));
#27156=DIRECTION('ref_axis',(-1.,0.,0.));
#27157=DIRECTION('center_axis',(0.,0.,1.));
#27158=DIRECTION('ref_axis',(1.,0.,0.));
#27159=DIRECTION('center_axis',(0.,0.,1.));
#27160=DIRECTION('ref_axis',(1.,0.,0.));
#27161=DIRECTION('',(0.,0.,-1.));
#27162=DIRECTION('center_axis',(0.,0.,-1.));
#27163=DIRECTION('ref_axis',(-1.,0.,0.));
#27164=DIRECTION('center_axis',(0.,0.,1.));
#27165=DIRECTION('ref_axis',(1.,0.,0.));
#27166=DIRECTION('center_axis',(0.,0.,1.));
#27167=DIRECTION('ref_axis',(1.,0.,0.));
#27168=DIRECTION('center_axis',(0.,0.,-1.));
#27169=DIRECTION('ref_axis',(-1.,1.22464679914735E-16,0.));
#27170=DIRECTION('center_axis',(1.22464679914735E-16,-1.,0.));
#27171=DIRECTION('ref_axis',(-1.,-1.22464679914735E-16,0.));
#27172=DIRECTION('center_axis',(0.,0.,1.));
#27173=DIRECTION('ref_axis',(-1.,0.,0.));
#27174=DIRECTION('center_axis',(0.,0.,1.));
#27175=DIRECTION('ref_axis',(1.,0.,0.));
#27176=DIRECTION('',(0.,0.,-1.));
#27177=DIRECTION('center_axis',(0.,0.,1.));
#27178=DIRECTION('ref_axis',(1.,0.,0.));
#27179=DIRECTION('',(0.821369965673296,1.00588809937757E-16,-0.570395809495344));
#27180=DIRECTION('center_axis',(0.,0.,1.));
#27181=DIRECTION('ref_axis',(1.,0.,0.));
#27182=DIRECTION('center_axis',(0.,0.,1.));
#27183=DIRECTION('ref_axis',(1.,0.,0.));
#27184=DIRECTION('center_axis',(0.,0.,1.));
#27185=DIRECTION('ref_axis',(1.,0.,0.));
#27186=DIRECTION('',(0.707106781186549,8.65956056235495E-17,-0.707106781186546));
#27187=DIRECTION('center_axis',(0.,0.,1.));
#27188=DIRECTION('ref_axis',(1.,0.,0.));
#27189=DIRECTION('',(0.,0.,-1.));
#27190=DIRECTION('center_axis',(0.,0.,1.));
#27191=DIRECTION('ref_axis',(1.,0.,0.));
#27192=DIRECTION('center_axis',(0.,0.,1.));
#27193=DIRECTION('ref_axis',(1.,0.,0.));
#27194=DIRECTION('',(0.707106781186547,8.65956056235492E-17,-0.707106781186548));
#27195=DIRECTION('center_axis',(0.,0.,1.));
#27196=DIRECTION('ref_axis',(1.,0.,0.));
#27197=DIRECTION('center_axis',(0.,0.,1.));
#27198=DIRECTION('ref_axis',(1.,0.,0.));
#27199=DIRECTION('',(0.,0.,-1.));
#27200=DIRECTION('center_axis',(0.,0.,-1.));
#27201=DIRECTION('ref_axis',(1.,0.,0.));
#27202=DIRECTION('',(-0.447213595499957,-5.47678698264201E-17,-0.894427190999917));
#27203=DIRECTION('center_axis',(0.,0.,1.));
#27204=DIRECTION('ref_axis',(1.,0.,0.));
#27205=DIRECTION('center_axis',(0.,0.,1.));
#27206=DIRECTION('ref_axis',(1.,0.,0.));
#27207=DIRECTION('center_axis',(0.,0.,1.));
#27208=DIRECTION('ref_axis',(1.,0.,0.));
#27209=DIRECTION('',(0.,0.,-1.));
#27210=DIRECTION('center_axis',(0.,0.,1.));
#27211=DIRECTION('ref_axis',(1.,0.,0.));
#27212=DIRECTION('center_axis',(0.,0.,1.));
#27213=DIRECTION('ref_axis',(1.,0.,0.));
#27214=DIRECTION('center_axis',(0.,0.,1.));
#27215=DIRECTION('ref_axis',(1.,0.,0.));
#27216=DIRECTION('center_axis',(0.,0.,1.));
#27217=DIRECTION('ref_axis',(1.,0.,0.));
#27218=DIRECTION('',(0.,0.,-1.));
#27219=DIRECTION('center_axis',(0.,0.,1.));
#27220=DIRECTION('ref_axis',(1.,0.,0.));
#27221=DIRECTION('center_axis',(0.,0.,-1.));
#27222=DIRECTION('ref_axis',(-1.,0.,0.));
#27223=DIRECTION('center_axis',(0.,0.,1.));
#27224=DIRECTION('ref_axis',(1.,0.,0.));
#27225=DIRECTION('center_axis',(0.,0.,1.));
#27226=DIRECTION('ref_axis',(1.,0.,0.));
#27227=DIRECTION('',(0.,0.,-1.));
#27228=DIRECTION('center_axis',(0.,0.,1.));
#27229=DIRECTION('ref_axis',(1.,0.,0.));
#27230=DIRECTION('center_axis',(0.,0.,1.));
#27231=DIRECTION('ref_axis',(1.,0.,0.));
#27232=DIRECTION('center_axis',(0.,0.,1.));
#27233=DIRECTION('ref_axis',(1.,0.,0.));
#27234=DIRECTION('center_axis',(0.,0.,1.));
#27235=DIRECTION('ref_axis',(1.,0.,0.));
#27236=DIRECTION('',(0.,0.,-1.));
#27237=DIRECTION('center_axis',(0.,0.,1.));
#27238=DIRECTION('ref_axis',(1.,0.,0.));
#27239=DIRECTION('center_axis',(0.,0.,1.));
#27240=DIRECTION('ref_axis',(1.,0.,0.));
#42303=CARTESIAN_POINT('',(0.,0.,0.));
#42304=CARTESIAN_POINT('Origin',(2.16374675043084,2.16374675043084,-12.4));
#42305=CARTESIAN_POINT('',(2.16374675043084,2.16374675043084,-12.4));
#42306=CARTESIAN_POINT('',(2.00818325856979,2.00818325856979,-12.4));
#42307=CARTESIAN_POINT('',(1.85687337521542,1.85687337521542,-12.4));
#42308=CARTESIAN_POINT('',(2.16374675043084,2.16374675043084,-12.36));
#42309=CARTESIAN_POINT('',(2.16374675043084,2.16374675043084,-12.4));
#42310=CARTESIAN_POINT('',(2.00818325856979,2.00818325856979,-12.36));
#42311=CARTESIAN_POINT('',(2.00818325856979,2.00818325856979,-12.36));
#42312=CARTESIAN_POINT('',(2.00818325856979,2.00818325856979,-12.4));
#42313=CARTESIAN_POINT('Origin',(2.33826859021798,1.35,-12.4));
#42314=CARTESIAN_POINT('',(2.33826859021798,1.35,-12.4));
#42315=CARTESIAN_POINT('',(2.49341599027072,0.62659086802724,-12.4));
#42316=CARTESIAN_POINT('',(2.33826859021798,1.35,-12.36));
#42317=CARTESIAN_POINT('',(2.33826859021798,1.35,-12.4));
#42318=CARTESIAN_POINT('',(2.16374675043084,2.16374675043084,-12.36));
#42319=CARTESIAN_POINT('Origin',(1.65462986797652,1.65462986797652,-12.4));
#42320=CARTESIAN_POINT('',(1.65462986797652,1.65462986797652,-12.4));
#42321=CARTESIAN_POINT('',(2.56517017788785,1.2488925020676,-12.4));
#42322=CARTESIAN_POINT('',(1.65462986797652,1.65462986797652,-12.36));
#42323=CARTESIAN_POINT('',(1.65462986797652,1.65462986797652,-12.4));
#42324=CARTESIAN_POINT('',(2.33826859021798,1.35,-12.36));
#42325=CARTESIAN_POINT('Origin',(1.81019335983756,1.81019335983756,-12.4));
#42326=CARTESIAN_POINT('',(1.81019335983756,1.81019335983756,-12.4));
#42327=CARTESIAN_POINT('',(1.68009667991878,1.68009667991878,-12.4));
#42328=CARTESIAN_POINT('',(1.81019335983756,1.81019335983756,-12.36));
#42329=CARTESIAN_POINT('',(1.81019335983756,1.81019335983756,-12.4));
#42330=CARTESIAN_POINT('',(1.65462986797652,1.65462986797652,-12.36));
#42331=CARTESIAN_POINT('Origin',(0.,-8.88178419700125E-16,-12.4));
#42332=CARTESIAN_POINT('',(-1.81019335983756,1.81019335983756,-12.4));
#42333=CARTESIAN_POINT('Origin',(0.,-8.88178419700125E-16,-12.4));
#42334=CARTESIAN_POINT('',(-1.81019335983756,1.81019335983756,-12.36));
#42335=CARTESIAN_POINT('',(-1.81019335983756,1.81019335983756,-12.4));
#42336=CARTESIAN_POINT('Origin',(0.,-8.88178419700125E-16,-12.36));
#42337=CARTESIAN_POINT('Origin',(-2.00818325856979,2.00818325856979,-12.4));
#42338=CARTESIAN_POINT('',(-2.00818325856979,2.00818325856979,-12.4));
#42339=CARTESIAN_POINT('',(-0.229091629284896,0.229091629284898,-12.4));
#42340=CARTESIAN_POINT('',(-2.00818325856979,2.00818325856979,-12.36));
#42341=CARTESIAN_POINT('',(-2.00818325856979,2.00818325856979,-12.4));
#42342=CARTESIAN_POINT('',(-1.81019335983756,1.81019335983756,-12.36));
#42343=CARTESIAN_POINT('Origin',(2.22044604925031E-16,4.44089209850063E-16,
-12.4));
#42344=CARTESIAN_POINT('Origin',(2.22044604925031E-16,4.44089209850063E-16,
-12.4));
#42345=CARTESIAN_POINT('Origin',(2.22044604925031E-16,4.44089209850063E-16,
-12.36));
#42346=CARTESIAN_POINT('Origin',(0.165042665824095,2.095,-12.36));
#42347=CARTESIAN_POINT('Origin',(6.,0.,-0.5275));
#42348=CARTESIAN_POINT('',(6.475,-5.81707229594993E-17,-0.54));
#42349=CARTESIAN_POINT('Origin',(6.,0.,-0.54));
#42350=CARTESIAN_POINT('',(6.45,5.51091059616309E-17,-0.515));
#42351=CARTESIAN_POINT('',(6.4625,-5.66399144605651E-17,-0.5275));
#42352=CARTESIAN_POINT('',(5.55,-5.51091059616309E-17,-0.515));
#42353=CARTESIAN_POINT('Origin',(6.,0.,-0.515));
#42354=CARTESIAN_POINT('Origin',(6.,0.,-0.515));
#42355=CARTESIAN_POINT('Origin',(6.45,0.,-0.54));
#42356=CARTESIAN_POINT('',(5.3,-8.57252759403147E-17,-0.54));
#42357=CARTESIAN_POINT('Origin',(6.,0.,-0.54));
#42358=CARTESIAN_POINT('Origin',(6.,0.,-0.22));
#42359=CARTESIAN_POINT('',(5.55,5.51091059616309E-17,0.));
#42360=CARTESIAN_POINT('',(5.55,-5.51091059616309E-17,-0.22));
#42361=CARTESIAN_POINT('Origin',(6.,0.,0.));
#42362=CARTESIAN_POINT('Origin',(3.,5.19615242270663,-0.5275));
#42363=CARTESIAN_POINT('',(3.475,5.19615242270663,-0.54));
#42364=CARTESIAN_POINT('Origin',(3.,5.19615242270663,-0.54));
#42365=CARTESIAN_POINT('',(3.45,5.19615242270663,-0.515));
#42366=CARTESIAN_POINT('',(3.4625,5.19615242270663,-0.5275));
#42367=CARTESIAN_POINT('',(2.55,5.19615242270663,-0.515));
#42368=CARTESIAN_POINT('Origin',(3.,5.19615242270663,-0.515));
#42369=CARTESIAN_POINT('Origin',(3.,5.19615242270663,-0.515));
#42370=CARTESIAN_POINT('Origin',(3.45,5.19615242270663,-0.54));
#42371=CARTESIAN_POINT('',(2.3,5.19615242270663,-0.54));
#42372=CARTESIAN_POINT('Origin',(3.,5.19615242270663,-0.54));
#42373=CARTESIAN_POINT('Origin',(3.,5.19615242270663,-0.22));
#42374=CARTESIAN_POINT('',(2.55,5.19615242270663,0.));
#42375=CARTESIAN_POINT('',(2.55,5.19615242270663,-0.22));
#42376=CARTESIAN_POINT('Origin',(3.,5.19615242270663,0.));
#42377=CARTESIAN_POINT('Origin',(-3.,5.19615242270663,-0.5275));
#42378=CARTESIAN_POINT('',(-2.525,5.19615242270663,-0.54));
#42379=CARTESIAN_POINT('Origin',(-3.,5.19615242270663,-0.54));
#42380=CARTESIAN_POINT('',(-2.55,5.19615242270663,-0.515));
#42381=CARTESIAN_POINT('',(-2.5375,5.19615242270663,-0.5275));
#42382=CARTESIAN_POINT('',(-3.45,5.19615242270663,-0.515));
#42383=CARTESIAN_POINT('Origin',(-3.,5.19615242270663,-0.515));
#42384=CARTESIAN_POINT('Origin',(-3.,5.19615242270663,-0.515));
#42385=CARTESIAN_POINT('Origin',(-2.55,5.19615242270663,-0.54));
#42386=CARTESIAN_POINT('',(-3.7,5.19615242270663,-0.54));
#42387=CARTESIAN_POINT('Origin',(-3.,5.19615242270663,-0.54));
#42388=CARTESIAN_POINT('Origin',(-3.,5.19615242270663,-0.22));
#42389=CARTESIAN_POINT('',(-3.45,5.19615242270663,0.));
#42390=CARTESIAN_POINT('',(-3.45,5.19615242270663,-0.22));
#42391=CARTESIAN_POINT('Origin',(-3.,5.19615242270663,0.));
#42392=CARTESIAN_POINT('Origin',(-6.,7.34788079488412E-16,-0.5275));
#42393=CARTESIAN_POINT('',(-5.525,6.76617356528913E-16,-0.54));
#42394=CARTESIAN_POINT('Origin',(-6.,7.34788079488412E-16,-0.54));
#42395=CARTESIAN_POINT('',(-5.55,7.89897185450043E-16,-0.515));
#42396=CARTESIAN_POINT('',(-5.5375,6.78148165027847E-16,-0.5275));
#42397=CARTESIAN_POINT('',(-6.45,6.79678973526781E-16,-0.515));
#42398=CARTESIAN_POINT('Origin',(-6.,7.34788079488412E-16,-0.515));
#42399=CARTESIAN_POINT('Origin',(-6.,7.34788079488412E-16,-0.515));
#42400=CARTESIAN_POINT('Origin',(-5.55,7.34788079488412E-16,-0.54));
#42401=CARTESIAN_POINT('',(-6.7,6.49062803548097E-16,-0.54));
#42402=CARTESIAN_POINT('Origin',(-6.,7.34788079488412E-16,-0.54));
#42403=CARTESIAN_POINT('Origin',(-6.,7.34788079488412E-16,-0.22));
#42404=CARTESIAN_POINT('',(-6.45,7.89897185450043E-16,0.));
#42405=CARTESIAN_POINT('',(-6.45,6.79678973526781E-16,-0.22));
#42406=CARTESIAN_POINT('Origin',(-6.,7.34788079488412E-16,0.));
#42407=CARTESIAN_POINT('Origin',(-3.,-5.19615242270663,-0.5275));
#42408=CARTESIAN_POINT('',(-2.525,-5.19615242270663,-0.54));
#42409=CARTESIAN_POINT('Origin',(-3.,-5.19615242270663,-0.54));
#42410=CARTESIAN_POINT('',(-2.55,-5.19615242270663,-0.515));
#42411=CARTESIAN_POINT('',(-2.5375,-5.19615242270663,-0.5275));
#42412=CARTESIAN_POINT('',(-3.45,-5.19615242270663,-0.515));
#42413=CARTESIAN_POINT('Origin',(-3.,-5.19615242270663,-0.515));
#42414=CARTESIAN_POINT('Origin',(-3.,-5.19615242270663,-0.515));
#42415=CARTESIAN_POINT('Origin',(-2.55,-5.19615242270663,-0.54));
#42416=CARTESIAN_POINT('',(-3.7,-5.19615242270663,-0.54));
#42417=CARTESIAN_POINT('Origin',(-3.,-5.19615242270663,-0.54));
#42418=CARTESIAN_POINT('Origin',(-3.,-5.19615242270663,-0.22));
#42419=CARTESIAN_POINT('',(-3.45,-5.19615242270663,0.));
#42420=CARTESIAN_POINT('',(-3.45,-5.19615242270663,-0.22));
#42421=CARTESIAN_POINT('Origin',(-3.,-5.19615242270663,0.));
#42422=CARTESIAN_POINT('Origin',(3.,-5.19615242270663,-0.5275));
#42423=CARTESIAN_POINT('',(3.475,-5.19615242270663,-0.54));
#42424=CARTESIAN_POINT('Origin',(3.,-5.19615242270663,-0.54));
#42425=CARTESIAN_POINT('',(3.45,-5.19615242270663,-0.515));
#42426=CARTESIAN_POINT('',(3.4625,-5.19615242270663,-0.5275));
#42427=CARTESIAN_POINT('',(2.55,-5.19615242270663,-0.515));
#42428=CARTESIAN_POINT('Origin',(3.,-5.19615242270663,-0.515));
#42429=CARTESIAN_POINT('Origin',(3.,-5.19615242270663,-0.515));
#42430=CARTESIAN_POINT('Origin',(3.45,-5.19615242270663,-0.54));
#42431=CARTESIAN_POINT('',(2.3,-5.19615242270663,-0.54));
#42432=CARTESIAN_POINT('Origin',(3.,-5.19615242270663,-0.54));
#42433=CARTESIAN_POINT('Origin',(3.,-5.19615242270663,-0.22));
#42434=CARTESIAN_POINT('',(2.55,-5.19615242270663,0.));
#42435=CARTESIAN_POINT('',(2.55,-5.19615242270663,-0.22));
#42436=CARTESIAN_POINT('Origin',(3.,-5.19615242270663,0.));
#42437=CARTESIAN_POINT('Origin',(3.,-5.19615242270663,-0.985));
#42438=CARTESIAN_POINT('',(2.398505676009,-4.83809575371888,-1.4));
#42439=CARTESIAN_POINT('',(2.3,-5.19615242270663,-1.4));
#42440=CARTESIAN_POINT('Origin',(3.,-5.19615242270663,-1.4));
#42441=CARTESIAN_POINT('',(2.99066099065767,-4.4962147234044,-1.4));
#42442=CARTESIAN_POINT('Ctrl Pts',(2.99066099065767,-4.4962147234044,-1.4));
#42443=CARTESIAN_POINT('Ctrl Pts',(2.94435268993459,-4.49683259790025,-1.4));
#42444=CARTESIAN_POINT('Ctrl Pts',(2.89813146126322,-4.50204848216744,-1.40231938147182));
#42445=CARTESIAN_POINT('Ctrl Pts',(2.81323479915933,-4.52031941214783,-1.40701255737455));
#42446=CARTESIAN_POINT('Ctrl Pts',(2.77447068348404,-4.53224035984442,-1.40932756283484));
#42447=CARTESIAN_POINT('Ctrl Pts',(2.71745752705182,-4.55536347077066,-1.41160495505446));
#42448=CARTESIAN_POINT('Ctrl Pts',(2.6983740351221,-4.56412140103041,-1.41217031646736));
#42449=CARTESIAN_POINT('Ctrl Pts',(2.66481875075551,-4.5813895902509,-1.41269782155031));
#42450=CARTESIAN_POINT('Ctrl Pts',(2.65023281412281,-4.58956955455007,-1.41275985502411));
#42451=CARTESIAN_POINT('Ctrl Pts',(2.6199950909463,-4.60798156330058,-1.41251886218627));
#42452=CARTESIAN_POINT('Ctrl Pts',(2.6044553894058,-4.61831783859573,-1.41217237294443));
#42453=CARTESIAN_POINT('Ctrl Pts',(2.5646618286732,-4.64714483808501,-1.41075856218782));
#42454=CARTESIAN_POINT('Ctrl Pts',(2.54121423306641,-4.66658595835824,-1.40936726373267));
#42455=CARTESIAN_POINT('Ctrl Pts',(2.47069726020893,-4.73325103677911,-1.40429573999265));
#42456=CARTESIAN_POINT('Ctrl Pts',(2.43054124554308,-4.78427965445435,-1.4));
#42457=CARTESIAN_POINT('Ctrl Pts',(2.398505676009,-4.83809575371887,-1.4));
#42458=CARTESIAN_POINT('Origin',(3.,-5.19615242270663,-1.4));
#42459=CARTESIAN_POINT('',(2.3,-5.19615242270663,-0.985));
#42460=CARTESIAN_POINT('Origin',(0.,0.,-1.8));
#42461=CARTESIAN_POINT('',(-5.,-6.12323399573677E-16,-1.8));
#42462=CARTESIAN_POINT('Origin',(0.,0.,-1.8));
#42463=CARTESIAN_POINT('',(-5.3,-6.34179542235909E-16,-1.41270166537926));
#42464=CARTESIAN_POINT('Origin',(-5.4,-6.61309271539571E-16,-1.8));
#42465=CARTESIAN_POINT('',(-5.38916666666667,0.341881030314489,-1.4));
#42466=CARTESIAN_POINT('Ctrl Pts',(-5.3,-6.09688915147857E-16,-1.41270166537926));
#42467=CARTESIAN_POINT('Ctrl Pts',(-5.3,0.00489840697065965,-1.41270166537926));
#42468=CARTESIAN_POINT('Ctrl Pts',(-5.30005141287727,0.00979759623850979,
-1.41268662310038));
#42469=CARTESIAN_POINT('Ctrl Pts',(-5.30057443545454,0.0347025480229719,
-1.41253403311749));
#42470=CARTESIAN_POINT('Ctrl Pts',(-5.30185082372053,0.0546596314022927,
-1.41215873854401));
#42471=CARTESIAN_POINT('Ctrl Pts',(-5.30735883827001,0.106087707237653,
-1.41062705709453));
#42472=CARTESIAN_POINT('Ctrl Pts',(-5.3128706815181,0.137315022342647,-1.40913458836236));
#42473=CARTESIAN_POINT('Ctrl Pts',(-5.33593994566315,0.230600777255617,
-1.4040421544805));
#42474=CARTESIAN_POINT('Ctrl Pts',(-5.35950446427729,0.288884050801338,
-1.4));
#42475=CARTESIAN_POINT('Ctrl Pts',(-5.38916666666667,0.341881030314486,
-1.4));
#42476=CARTESIAN_POINT('',(-2.99066099065768,4.49621472340439,-1.4));
#42477=CARTESIAN_POINT('Origin',(0.,0.,-1.4));
#42478=CARTESIAN_POINT('',(-2.39850567600899,4.83809575371888,-1.4));
#42479=CARTESIAN_POINT('Ctrl Pts',(-2.99066099065768,4.4962147234044,-1.4));
#42480=CARTESIAN_POINT('Ctrl Pts',(-2.9443526899346,4.49683259790024,-1.4));
#42481=CARTESIAN_POINT('Ctrl Pts',(-2.89813146126323,4.50204848216743,-1.40231938147182));
#42482=CARTESIAN_POINT('Ctrl Pts',(-2.81323479915932,4.52031941214783,-1.40701255737455));
#42483=CARTESIAN_POINT('Ctrl Pts',(-2.77447068348403,4.53224035984442,-1.40932756283484));
#42484=CARTESIAN_POINT('Ctrl Pts',(-2.71745752705178,4.55536347077068,-1.41160495505446));
#42485=CARTESIAN_POINT('Ctrl Pts',(-2.69837403512208,4.56412140103042,-1.41217031646737));
#42486=CARTESIAN_POINT('Ctrl Pts',(-2.66481875075553,4.58138959025089,-1.41269782155031));
#42487=CARTESIAN_POINT('Ctrl Pts',(-2.65023281412282,4.58956955455007,-1.41275985502411));
#42488=CARTESIAN_POINT('Ctrl Pts',(-2.61999509094628,4.60798156330059,-1.41251886218627));
#42489=CARTESIAN_POINT('Ctrl Pts',(-2.60445538940576,4.61831783859576,-1.41217237294442));
#42490=CARTESIAN_POINT('Ctrl Pts',(-2.56466182867321,4.64714483808501,-1.41075856218782));
#42491=CARTESIAN_POINT('Ctrl Pts',(-2.54121423306642,4.66658595835823,-1.40936726373267));
#42492=CARTESIAN_POINT('Ctrl Pts',(-2.47069726020893,4.73325103677911,-1.40429573999265));
#42493=CARTESIAN_POINT('Ctrl Pts',(-2.43054124554308,4.78427965445436,-1.4));
#42494=CARTESIAN_POINT('Ctrl Pts',(-2.39850567600899,4.83809575371888,-1.4));
#42495=CARTESIAN_POINT('',(2.398505676009,4.83809575371888,-1.4));
#42496=CARTESIAN_POINT('Origin',(0.,0.,-1.4));
#42497=CARTESIAN_POINT('',(2.99066099065767,4.4962147234044,-1.4));
#42498=CARTESIAN_POINT('Ctrl Pts',(2.398505676009,4.83809575371888,-1.4));
#42499=CARTESIAN_POINT('Ctrl Pts',(2.42219492138029,4.79830052613452,-1.4));
#42500=CARTESIAN_POINT('Ctrl Pts',(2.44982262399457,4.76087971004458,-1.40231938147182));
#42501=CARTESIAN_POINT('Ctrl Pts',(2.5080940445603,4.69649250895631,-1.40701255737455));
#42502=CARTESIAN_POINT('Ctrl Pts',(2.53779994594037,4.66888227387456,-1.40932756283484));
#42503=CARTESIAN_POINT('Ctrl Pts',(2.58633172563316,4.63106898751742,-1.41160495505446));
#42504=CARTESIAN_POINT('Ctrl Pts',(2.60345806168753,4.61892116384326,-1.41217031646736));
#42505=CARTESIAN_POINT('Ctrl Pts',(2.63519039441309,4.59849552976084,-1.41269782155031));
#42506=CARTESIAN_POINT('Ctrl Pts',(2.64956741961458,4.58995372024851,-1.41275985502411));
#42507=CARTESIAN_POINT('Ctrl Pts',(2.6806315485155,4.5729730882003,-1.41251886218627));
#42508=CARTESIAN_POINT('Ctrl Pts',(2.69735287627189,4.56468344954656,-1.41217237294442));
#42509=CARTESIAN_POINT('Ctrl Pts',(2.74221457051073,4.54463471478976,-1.41075856218782));
#42510=CARTESIAN_POINT('Ctrl Pts',(2.77077487234875,4.53404906147323,-1.40936726373267));
#42511=CARTESIAN_POINT('Ctrl Pts',(2.86376701023529,4.5063121107911,-1.40429573999265));
#42512=CARTESIAN_POINT('Ctrl Pts',(2.92803709679497,4.49705029081335,-1.4));
#42513=CARTESIAN_POINT('Ctrl Pts',(2.99066099065767,4.4962147234044,-1.4));
#42514=CARTESIAN_POINT('',(5.38916666666667,0.341881030314488,-1.4));
#42515=CARTESIAN_POINT('Origin',(0.,0.,-1.4));
#42516=CARTESIAN_POINT('',(5.3,-7.14855753237747E-17,-1.41270166537926));
#42517=CARTESIAN_POINT('Ctrl Pts',(5.38916666666667,0.341881030314486,-1.4));
#42518=CARTESIAN_POINT('Ctrl Pts',(5.37147004253223,0.310262756850054,-1.4));
#42519=CARTESIAN_POINT('Ctrl Pts',(5.35620231261546,0.277219041062471,-1.40143366869053));
#42520=CARTESIAN_POINT('Ctrl Pts',(5.32761567846875,0.200017956511915,-1.40554873470576));
#42521=CARTESIAN_POINT('Ctrl Pts',(5.31589717989396,0.155336805463026,-1.40841107882748));
#42522=CARTESIAN_POINT('Ctrl Pts',(5.30499765049498,0.086708007070014,-1.4112618373153));
#42523=CARTESIAN_POINT('Ctrl Pts',(5.30248948591046,0.0634567556288577,
-1.41198187968474));
#42524=CARTESIAN_POINT('Ctrl Pts',(5.300382961066,0.0267381544766715,-1.41258893738177));
#42525=CARTESIAN_POINT('Ctrl Pts',(5.3,0.0133719921338023,-1.41270166537926));
#42526=CARTESIAN_POINT('Ctrl Pts',(5.3,-4.5102810375397E-17,-1.41270166537926));
#42527=CARTESIAN_POINT('',(5.38916666666667,-0.341881030314488,-1.4));
#42528=CARTESIAN_POINT('Ctrl Pts',(5.3,-4.60309413329061E-17,-1.41270166537926));
#42529=CARTESIAN_POINT('Ctrl Pts',(5.3,-0.00489840697065912,-1.41270166537926));
#42530=CARTESIAN_POINT('Ctrl Pts',(5.30005141287727,-0.00979759623850861,
-1.41268662310038));
#42531=CARTESIAN_POINT('Ctrl Pts',(5.30057443545454,-0.0347025480229614,
-1.41253403311749));
#42532=CARTESIAN_POINT('Ctrl Pts',(5.30185082372053,-0.0546596314022734,
-1.41215873854401));
#42533=CARTESIAN_POINT('Ctrl Pts',(5.30735883827001,-0.10608770723766,-1.41062705709453));
#42534=CARTESIAN_POINT('Ctrl Pts',(5.31287068151811,-0.137315022342663,
-1.40913458836236));
#42535=CARTESIAN_POINT('Ctrl Pts',(5.33593994566315,-0.230600777255612,
-1.4040421544805));
#42536=CARTESIAN_POINT('Ctrl Pts',(5.35950446427729,-0.288884050801334,
-1.4));
#42537=CARTESIAN_POINT('Ctrl Pts',(5.38916666666667,-0.341881030314486,
-1.4));
#42538=CARTESIAN_POINT('Origin',(0.,0.,-1.4));
#42539=CARTESIAN_POINT('',(-2.398505676009,-4.83809575371888,-1.4));
#42540=CARTESIAN_POINT('Origin',(0.,0.,-1.4));
#42541=CARTESIAN_POINT('',(-2.99066099065767,-4.4962147234044,-1.4));
#42542=CARTESIAN_POINT('Ctrl Pts',(-2.398505676009,-4.83809575371888,-1.4));
#42543=CARTESIAN_POINT('Ctrl Pts',(-2.4221949213803,-4.79830052613452,-1.4));
#42544=CARTESIAN_POINT('Ctrl Pts',(-2.44982262399457,-4.76087971004458,
-1.40231938147182));
#42545=CARTESIAN_POINT('Ctrl Pts',(-2.5080940445603,-4.6964925089563,-1.40701255737455));
#42546=CARTESIAN_POINT('Ctrl Pts',(-2.53779994594038,-4.66888227387456,
-1.40932756283484));
#42547=CARTESIAN_POINT('Ctrl Pts',(-2.58633172563316,-4.63106898751742,
-1.41160495505446));
#42548=CARTESIAN_POINT('Ctrl Pts',(-2.60345806168753,-4.61892116384326,
-1.41217031646736));
#42549=CARTESIAN_POINT('Ctrl Pts',(-2.6351903944131,-4.59849552976084,-1.41269782155031));
#42550=CARTESIAN_POINT('Ctrl Pts',(-2.64956741961458,-4.58995372024851,
-1.41275985502411));
#42551=CARTESIAN_POINT('Ctrl Pts',(-2.6806315485155,-4.5729730882003,-1.41251886218627));
#42552=CARTESIAN_POINT('Ctrl Pts',(-2.69735287627188,-4.56468344954657,
-1.41217237294442));
#42553=CARTESIAN_POINT('Ctrl Pts',(-2.74221457051074,-4.54463471478975,
-1.41075856218782));
#42554=CARTESIAN_POINT('Ctrl Pts',(-2.77077487234877,-4.53404906147323,
-1.40936726373267));
#42555=CARTESIAN_POINT('Ctrl Pts',(-2.86376701023528,-4.5063121107911,-1.40429573999265));
#42556=CARTESIAN_POINT('Ctrl Pts',(-2.92803709679497,-4.49705029081335,
-1.4));
#42557=CARTESIAN_POINT('Ctrl Pts',(-2.99066099065767,-4.4962147234044,-1.4));
#42558=CARTESIAN_POINT('',(-5.38916666666667,-0.341881030314487,-1.4));
#42559=CARTESIAN_POINT('Origin',(0.,0.,-1.4));
#42560=CARTESIAN_POINT('Ctrl Pts',(-5.38916666666667,-0.341881030314485,
-1.4));
#42561=CARTESIAN_POINT('Ctrl Pts',(-5.37147004253223,-0.310262756850051,
-1.4));
#42562=CARTESIAN_POINT('Ctrl Pts',(-5.35620231261545,-0.277219041062467,
-1.40143366869053));
#42563=CARTESIAN_POINT('Ctrl Pts',(-5.32761567846876,-0.200017956511921,
-1.40554873470576));
#42564=CARTESIAN_POINT('Ctrl Pts',(-5.31589717989396,-0.155336805463029,
-1.40841107882748));
#42565=CARTESIAN_POINT('Ctrl Pts',(-5.30499765049498,-0.0867080070700145,
-1.4112618373153));
#42566=CARTESIAN_POINT('Ctrl Pts',(-5.30248948591046,-0.0634567556288565,
-1.41198187968474));
#42567=CARTESIAN_POINT('Ctrl Pts',(-5.300382961066,-0.0267381544766586,
-1.41258893738177));
#42568=CARTESIAN_POINT('Ctrl Pts',(-5.3,-0.0133719921337942,-1.41270166537926));
#42569=CARTESIAN_POINT('Ctrl Pts',(-5.3,-6.1409211049579E-16,-1.41270166537926));
#42570=CARTESIAN_POINT('Origin',(-3.,-5.19615242270663,-0.985));
#42571=CARTESIAN_POINT('',(-3.7,-5.19615242270663,-1.4));
#42572=CARTESIAN_POINT('Origin',(-3.,-5.19615242270663,-1.4));
#42573=CARTESIAN_POINT('',(-3.7,-5.19615242270663,-0.985));
#42574=CARTESIAN_POINT('Origin',(-3.,-5.19615242270663,-1.4));
#42575=CARTESIAN_POINT('Origin',(6.9,0.,-1.4));
#42576=CARTESIAN_POINT('',(-6.9,-8.45006291411674E-16,-1.4));
#42577=CARTESIAN_POINT('Origin',(0.,0.,-1.4));
#42578=CARTESIAN_POINT('Origin',(6.,0.,-1.4));
#42579=CARTESIAN_POINT('',(2.3,5.19615242270663,-1.4));
#42580=CARTESIAN_POINT('Origin',(3.,5.19615242270663,-1.4));
#42581=CARTESIAN_POINT('Origin',(3.,5.19615242270663,-1.4));
#42582=CARTESIAN_POINT('',(-3.7,5.19615242270663,-1.4));
#42583=CARTESIAN_POINT('Origin',(-3.,5.19615242270663,-1.4));
#42584=CARTESIAN_POINT('Origin',(-3.,5.19615242270663,-1.4));
#42585=CARTESIAN_POINT('',(-6.7,6.49062803548097E-16,-1.4));
#42586=CARTESIAN_POINT('Origin',(-6.,7.34788079488412E-16,-1.4));
#42587=CARTESIAN_POINT('Origin',(-6.,7.34788079488412E-16,-1.4));
#42588=CARTESIAN_POINT('Origin',(-6.,7.34788079488412E-16,-0.985));
#42589=CARTESIAN_POINT('',(-6.7,6.49062803548097E-16,-0.985));
#42590=CARTESIAN_POINT('Origin',(-3.,5.19615242270663,-0.985));
#42591=CARTESIAN_POINT('',(-3.7,5.19615242270663,-0.985));
#42592=CARTESIAN_POINT('Origin',(3.,5.19615242270663,-0.985));
#42593=CARTESIAN_POINT('',(2.3,5.19615242270663,-0.985));
#42594=CARTESIAN_POINT('Origin',(6.,0.,-0.985));
#42595=CARTESIAN_POINT('',(5.3,-8.57252759403147E-17,-0.985));
#42596=CARTESIAN_POINT('Origin',(5.16,0.,-4.));
#42597=CARTESIAN_POINT('',(5.2,9.09728874746612E-17,-4.74285));
#42598=CARTESIAN_POINT('Origin',(5.2,0.,-4.));
#42599=CARTESIAN_POINT('',(5.12,-8.11757130814823E-17,-4.66285));
#42600=CARTESIAN_POINT('',(5.16,8.60743002780717E-17,-4.70285));
#42601=CARTESIAN_POINT('Origin',(5.12,0.,-4.));
#42602=CARTESIAN_POINT('Origin',(4.615,0.,-4.));
#42603=CARTESIAN_POINT('',(4.3,-9.6099007771999E-17,-4.66285));
#42604=CARTESIAN_POINT('',(4.615,-8.11757130814823E-17,-4.66285));
#42605=CARTESIAN_POINT('',(4.24860328549277,-0.66285,-4.));
#42606=CARTESIAN_POINT('Ctrl Pts',(4.24860328549277,-0.66285,-4.));
#42607=CARTESIAN_POINT('Ctrl Pts',(4.24860328549277,-0.66285,-4.08337270554936));
#42608=CARTESIAN_POINT('Ctrl Pts',(4.25131103029984,-0.646160681103361,
-4.17221014517061));
#42609=CARTESIAN_POINT('Ctrl Pts',(4.26104887749279,-0.578473468430526,
-4.33548236983766));
#42610=CARTESIAN_POINT('Ctrl Pts',(4.26793372257373,-0.527482714273786,
-4.40992874554522));
#42611=CARTESIAN_POINT('Ctrl Pts',(4.28082394210211,-0.409929889997929,
-4.52748156982108));
#42612=CARTESIAN_POINT('Ctrl Pts',(4.28767291694093,-0.335483021085273,
-4.57847322173307));
#42613=CARTESIAN_POINT('Ctrl Pts',(4.29732846342061,-0.172209109236183,
-4.64616108727907));
#42614=CARTESIAN_POINT('Ctrl Pts',(4.3,-0.0833710821908396,-4.66285));
#42615=CARTESIAN_POINT('Ctrl Pts',(4.3,-5.55111512312578E-17,-4.66285));
#42616=CARTESIAN_POINT('Ctrl Pts',(4.3,-1.11022302462516E-16,-4.66285));
#42617=CARTESIAN_POINT('Ctrl Pts',(4.3,0.0833710821908394,-4.66285));
#42618=CARTESIAN_POINT('Ctrl Pts',(4.29732846342061,0.172209109236183,-4.64616108727907));
#42619=CARTESIAN_POINT('Ctrl Pts',(4.28767291694093,0.335483021085273,-4.57847322173307));
#42620=CARTESIAN_POINT('Ctrl Pts',(4.28082394210211,0.409929889997929,-4.52748156982108));
#42621=CARTESIAN_POINT('Ctrl Pts',(4.26793372257373,0.527482714273785,-4.40992874554522));
#42622=CARTESIAN_POINT('Ctrl Pts',(4.26104887749279,0.578473468430526,-4.33548236983766));
#42623=CARTESIAN_POINT('Ctrl Pts',(4.25131103029984,0.646160681103361,-4.17221014517061));
#42624=CARTESIAN_POINT('Ctrl Pts',(4.24860328549277,0.66285,-4.08337270554937));
#42625=CARTESIAN_POINT('Ctrl Pts',(4.24860328549277,0.66285,-3.91662729445063));
#42626=CARTESIAN_POINT('Ctrl Pts',(4.25131103029984,0.646160681103361,-3.82778985482939));
#42627=CARTESIAN_POINT('Ctrl Pts',(4.26104887749279,0.578473468430526,-3.66451763016234));
#42628=CARTESIAN_POINT('Ctrl Pts',(4.26793372257373,0.527482714273786,-3.59007125445478));
#42629=CARTESIAN_POINT('Ctrl Pts',(4.28082394210211,0.40992988999793,-3.47251843017892));
#42630=CARTESIAN_POINT('Ctrl Pts',(4.28767291694093,0.335483021085274,-3.42152677826693));
#42631=CARTESIAN_POINT('Ctrl Pts',(4.29732846342061,0.172209109236183,-3.35383891272093));
#42632=CARTESIAN_POINT('Ctrl Pts',(4.3,0.0833710821908397,-3.33715));
#42633=CARTESIAN_POINT('Ctrl Pts',(4.3,-0.0833710821908394,-3.33715));
#42634=CARTESIAN_POINT('Ctrl Pts',(4.29732846342061,-0.172209109236183,
-3.35383891272093));
#42635=CARTESIAN_POINT('Ctrl Pts',(4.28767291694093,-0.335483021085273,
-3.42152677826693));
#42636=CARTESIAN_POINT('Ctrl Pts',(4.28082394210211,-0.409929889997929,
-3.47251843017892));
#42637=CARTESIAN_POINT('Ctrl Pts',(4.26793372257373,-0.527482714273785,
-3.59007125445478));
#42638=CARTESIAN_POINT('Ctrl Pts',(4.26104887749279,-0.578473468430526,
-3.66451763016234));
#42639=CARTESIAN_POINT('Ctrl Pts',(4.25131103029984,-0.646160681103361,
-3.82778985482939));
#42640=CARTESIAN_POINT('Ctrl Pts',(4.24860328549277,-0.66285,-3.91662729445063));
#42641=CARTESIAN_POINT('Ctrl Pts',(4.24860328549277,-0.66285,-4.));
#42642=CARTESIAN_POINT('Origin',(5.2,0.,-4.));
#42643=CARTESIAN_POINT('',(5.2,1.46957615897682E-16,-2.8));
#42644=CARTESIAN_POINT('Origin',(5.2,0.,-4.));
#42645=CARTESIAN_POINT('Origin',(5.15,0.,-4.));
#42646=CARTESIAN_POINT('',(5.1,-1.59204083889156E-16,-2.7));
#42647=CARTESIAN_POINT('',(5.15,-1.53080849893419E-16,-2.75));
#42648=CARTESIAN_POINT('Origin',(5.1,0.,-4.));
#42649=CARTESIAN_POINT('Origin',(4.4,0.,-4.));
#42650=CARTESIAN_POINT('',(5.,-1.62868768791465E-16,-2.7));
#42651=CARTESIAN_POINT('',(4.4,-1.59204083889156E-16,-2.7));
#42652=CARTESIAN_POINT('',(4.82804308182932,1.3,-4.));
#42653=CARTESIAN_POINT('Ctrl Pts',(4.82804308182932,1.3,-4.));
#42654=CARTESIAN_POINT('Ctrl Pts',(4.82804308182932,1.3,-4.16405971768551));
#42655=CARTESIAN_POINT('Ctrl Pts',(4.83727716857535,1.26705769140541,-4.33850900708893));
#42656=CARTESIAN_POINT('Ctrl Pts',(4.87015028662769,1.13416120781459,-4.65856059831929));
#42657=CARTESIAN_POINT('Ctrl Pts',(4.89326334703746,1.03424511530045,-4.80423251578458));
#42658=CARTESIAN_POINT('Ctrl Pts',(4.93628041072499,0.804251421167127,-5.0342262099179));
#42659=CARTESIAN_POINT('Ctrl Pts',(4.95904761708503,0.658571665059363,-5.1341570251573));
#42660=CARTESIAN_POINT('Ctrl Pts',(4.99112141383552,0.338492152411535,-5.26706427740736));
#42661=CARTESIAN_POINT('Ctrl Pts',(5.,0.164032748626163,-5.3));
#42662=CARTESIAN_POINT('Ctrl Pts',(5.,-0.164032748626163,-5.3));
#42663=CARTESIAN_POINT('Ctrl Pts',(4.99112141383552,-0.338492152411536,
-5.26706427740737));
#42664=CARTESIAN_POINT('Ctrl Pts',(4.95904761708503,-0.658571665059363,
-5.1341570251573));
#42665=CARTESIAN_POINT('Ctrl Pts',(4.93628041072499,-0.804251421167127,
-5.0342262099179));
#42666=CARTESIAN_POINT('Ctrl Pts',(4.89326334703746,-1.03424511530045,-4.80423251578458));
#42667=CARTESIAN_POINT('Ctrl Pts',(4.87015028662769,-1.13416120781459,-4.65856059831929));
#42668=CARTESIAN_POINT('Ctrl Pts',(4.83727716857535,-1.26705769140541,-4.33850900708893));
#42669=CARTESIAN_POINT('Ctrl Pts',(4.82804308182932,-1.3,-4.16405971768551));
#42670=CARTESIAN_POINT('Ctrl Pts',(4.82804308182932,-1.3,-3.83594028231449));
#42671=CARTESIAN_POINT('Ctrl Pts',(4.83727716857535,-1.26705769140541,-3.66149099291107));
#42672=CARTESIAN_POINT('Ctrl Pts',(4.87015028662769,-1.13416120781459,-3.34143940168072));
#42673=CARTESIAN_POINT('Ctrl Pts',(4.89326334703746,-1.03424511530045,-3.19576748421542));
#42674=CARTESIAN_POINT('Ctrl Pts',(4.93628041072499,-0.804251421167127,
-2.9657737900821));
#42675=CARTESIAN_POINT('Ctrl Pts',(4.95904761708503,-0.658571665059362,
-2.8658429748427));
#42676=CARTESIAN_POINT('Ctrl Pts',(4.99112141383552,-0.338492152411535,
-2.73293572259264));
#42677=CARTESIAN_POINT('Ctrl Pts',(5.,-0.164032748626163,-2.7));
#42678=CARTESIAN_POINT('Ctrl Pts',(5.,-2.22044604925031E-16,-2.7));
#42679=CARTESIAN_POINT('Ctrl Pts',(5.,-1.66533453693773E-16,-2.7));
#42680=CARTESIAN_POINT('Ctrl Pts',(5.,0.164032748626162,-2.7));
#42681=CARTESIAN_POINT('Ctrl Pts',(4.99112141383552,0.338492152411535,-2.73293572259263));
#42682=CARTESIAN_POINT('Ctrl Pts',(4.95904761708503,0.658571665059362,-2.8658429748427));
#42683=CARTESIAN_POINT('Ctrl Pts',(4.93628041072499,0.804251421167127,-2.9657737900821));
#42684=CARTESIAN_POINT('Ctrl Pts',(4.89326334703746,1.03424511530045,-3.19576748421542));
#42685=CARTESIAN_POINT('Ctrl Pts',(4.87015028662769,1.13416120781459,-3.34143940168072));
#42686=CARTESIAN_POINT('Ctrl Pts',(4.83727716857535,1.26705769140541,-3.66149099291107));
#42687=CARTESIAN_POINT('Ctrl Pts',(4.82804308182932,1.3,-3.83594028231449));
#42688=CARTESIAN_POINT('Ctrl Pts',(4.82804308182932,1.3,-4.));
#42689=CARTESIAN_POINT('Origin',(0.,0.,-0.0249999999999999));
#42690=CARTESIAN_POINT('',(4.3,-5.26598123633362E-16,-0.0499999999999998));
#42691=CARTESIAN_POINT('',(-4.3,-5.26598123633362E-16,-0.0499999999999998));
#42692=CARTESIAN_POINT('Origin',(0.,0.,-0.0499999999999998));
#42693=CARTESIAN_POINT('Origin',(0.,0.,-0.0499999999999998));
#42694=CARTESIAN_POINT('',(4.35,5.32721357629099E-16,0.));
#42695=CARTESIAN_POINT('',(4.325,-5.2965974063123E-16,-0.0249999999999999));
#42696=CARTESIAN_POINT('Origin',(0.,0.,0.));
#42697=CARTESIAN_POINT('Origin',(4.3,0.,0.));
#42698=CARTESIAN_POINT('',(-6.95,-8.5112952540741E-16,-3.19189119579733E-16));
#42699=CARTESIAN_POINT('Origin',(0.,0.,0.));
#42700=CARTESIAN_POINT('Origin',(0.,0.,-2.9));
#42701=CARTESIAN_POINT('',(-4.3,-5.26598123633362E-16,-5.8));
#42702=CARTESIAN_POINT('',(-4.3,-5.26598123633362E-16,-2.9));
#42703=CARTESIAN_POINT('Origin',(0.,0.,-5.8));
#42704=CARTESIAN_POINT('Origin',(0.,0.,-12.35));
#42705=CARTESIAN_POINT('',(2.1,-2.57175827820944E-16,-12.4));
#42706=CARTESIAN_POINT('Origin',(0.,0.,-12.4));
#42707=CARTESIAN_POINT('',(2.,2.44929359829471E-16,-12.3));
#42708=CARTESIAN_POINT('',(2.05,-2.51052593825207E-16,-12.35));
#42709=CARTESIAN_POINT('',(-2.,-2.44929359829471E-16,-12.3));
#42710=CARTESIAN_POINT('Origin',(0.,0.,-12.3));
#42711=CARTESIAN_POINT('Origin',(0.,0.,-12.3));
#42712=CARTESIAN_POINT('Origin',(0.,0.,-12.025));
#42713=CARTESIAN_POINT('',(-2.,-2.44929359829471E-16,-11.65));
#42714=CARTESIAN_POINT('Origin',(0.,0.,-11.65));
#42715=CARTESIAN_POINT('',(-2.,-2.44929359829471E-16,-12.025));
#42716=CARTESIAN_POINT('Origin',(3.1,0.,-12.4));
#42717=CARTESIAN_POINT('',(-3.1,-3.7964050773568E-16,-12.4));
#42718=CARTESIAN_POINT('Origin',(0.,0.,-12.4));
#42719=CARTESIAN_POINT('Origin',(0.,0.,-8.63617976663963));
#42720=CARTESIAN_POINT('',(-5.,-6.12323399573677E-16,-8.63617976663963));
#42721=CARTESIAN_POINT('Origin',(0.,0.,-8.63617976663963));
#42722=CARTESIAN_POINT('',(-4.74223748569721,-5.80756595765568E-16,-9.12900174604361));
#42723=CARTESIAN_POINT('Origin',(-4.4,-5.38844591624835E-16,-8.63617976663963));
#42724=CARTESIAN_POINT('Origin',(0.,-5.80756595765568E-16,-9.12900174604361));
#42725=CARTESIAN_POINT('Origin',(0.,0.,-5.175));
#42726=CARTESIAN_POINT('',(-5.,-6.12323399573677E-16,-5.175));
#42727=CARTESIAN_POINT('Origin',(0.,0.,-9.575));
#42728=CARTESIAN_POINT('',(-3.2,-3.91886975727153E-16,-10.2));
#42729=CARTESIAN_POINT('',(-4.1,-5.02105187650415E-16,-9.575));
#42730=CARTESIAN_POINT('Origin',(0.,0.,-10.2));
#42731=CARTESIAN_POINT('Origin',(0.,0.,-12.35));
#42732=CARTESIAN_POINT('',(-3.2,-3.91886975727153E-16,-12.3));
#42733=CARTESIAN_POINT('Origin',(0.,0.,-12.3));
#42734=CARTESIAN_POINT('',(-3.15,-3.85763741731416E-16,-12.35));
#42735=CARTESIAN_POINT('Origin',(0.,0.,-11.25));
#42736=CARTESIAN_POINT('',(-3.2,-3.91886975727153E-16,-11.25));
#42737=CARTESIAN_POINT('Origin',(0.,0.,-1.35));
#42738=CARTESIAN_POINT('',(-7.,-8.57252759403147E-16,-1.3));
#42739=CARTESIAN_POINT('Origin',(0.,0.,-1.3));
#42740=CARTESIAN_POINT('',(-6.95,-8.51129525407411E-16,-1.35));
#42741=CARTESIAN_POINT('Origin',(0.,0.,-0.699999999999999));
#42742=CARTESIAN_POINT('',(-7.,-8.57252759403147E-16,-0.0999999999999996));
#42743=CARTESIAN_POINT('Origin',(0.,0.,-0.0999999999999996));
#42744=CARTESIAN_POINT('',(-7.,-8.57252759403147E-16,-0.699999999999999));
#42745=CARTESIAN_POINT('Origin',(0.,0.,-0.0500000000000007));
#42746=CARTESIAN_POINT('',(-6.975,-8.54191142405279E-16,-0.0500000000000007));
#42747=CARTESIAN_POINT('Origin',(4.005,0.,-5.8));
#42748=CARTESIAN_POINT('',(-4.005,-4.90471043058515E-16,-5.8));
#42749=CARTESIAN_POINT('Origin',(0.,0.,-5.8));
#42750=CARTESIAN_POINT('Origin',(0.,0.,-7.5));
#42751=CARTESIAN_POINT('',(-4.005,-4.90471043058515E-16,-9.2));
#42752=CARTESIAN_POINT('',(-4.005,-4.90471043058515E-16,-7.5));
#42753=CARTESIAN_POINT('Origin',(0.,0.,-9.2));
#42754=CARTESIAN_POINT('Origin',(2.2,0.,-9.2));
#42755=CARTESIAN_POINT('',(-2.2,-2.69422295812418E-16,-9.2));
#42756=CARTESIAN_POINT('Origin',(0.,0.,-9.2));
#42757=CARTESIAN_POINT('Origin',(0.,0.,-9.4));
#42758=CARTESIAN_POINT('',(-2.2,-2.69422295812418E-16,-9.6));
#42759=CARTESIAN_POINT('',(-2.2,-2.69422295812418E-16,-9.4));
#42760=CARTESIAN_POINT('Origin',(0.,0.,-9.6));
#42761=CARTESIAN_POINT('Origin',(2.6,0.,-9.6));
#42762=CARTESIAN_POINT('',(-2.6,-3.18408167778312E-16,-9.6));
#42763=CARTESIAN_POINT('Origin',(0.,0.,-9.6));
#42764=CARTESIAN_POINT('Origin',(0.,0.,-10.25));
#42765=CARTESIAN_POINT('',(-2.6,-3.18408167778312E-16,-10.9));
#42766=CARTESIAN_POINT('',(-2.6,-3.18408167778312E-16,-10.25));
#42767=CARTESIAN_POINT('Origin',(0.,0.,-10.9));
#42768=CARTESIAN_POINT('Origin',(2.4,0.,-10.9));
#42769=CARTESIAN_POINT('',(-2.4,-2.93915231795365E-16,-10.9));
#42770=CARTESIAN_POINT('Origin',(0.,0.,-10.9));
#42771=CARTESIAN_POINT('Origin',(0.,0.,-11.275));
#42772=CARTESIAN_POINT('',(-2.4,-2.93915231795365E-16,-11.65));
#42773=CARTESIAN_POINT('',(-2.4,-2.93915231795365E-16,-11.275));
#42774=CARTESIAN_POINT('Origin',(0.,0.,-11.65));
#42775=CARTESIAN_POINT('Origin',(2.,0.,-11.65));
#59172=UNCERTAINTY_MEASURE_WITH_UNIT(LENGTH_MEASURE(0.001),#59205,
'DISTANCE_ACCURACY_VALUE',
'Maximum model space distance between geometric entities at asserted c
onnectivities');
#59182=UNCERTAINTY_MEASURE_WITH_UNIT(LENGTH_MEASURE(0.001),#59205,
'DISTANCE_ACCURACY_VALUE',
'Maximum model space distance between geometric entities at asserted c
onnectivities');
#59194=(
GEOMETRIC_REPRESENTATION_CONTEXT(3)
GLOBAL_UNCERTAINTY_ASSIGNED_CONTEXT((#59172))
GLOBAL_UNIT_ASSIGNED_CONTEXT((#59205,#59207,#59208))
REPRESENTATION_CONTEXT('','3D')
);
#59204=(
GEOMETRIC_REPRESENTATION_CONTEXT(3)
GLOBAL_UNCERTAINTY_ASSIGNED_CONTEXT((#59182))
GLOBAL_UNIT_ASSIGNED_CONTEXT((#59205,#59207,#59208))
REPRESENTATION_CONTEXT('','3D')
);
#59205=(
LENGTH_UNIT()
NAMED_UNIT(*)
SI_UNIT(.CENTI.,.METRE.)
);
#59207=(
NAMED_UNIT(*)
PLANE_ANGLE_UNIT()
SI_UNIT($,.RADIAN.)
);
#59208=(
NAMED_UNIT(*)
SI_UNIT($,.STERADIAN.)
SOLID_ANGLE_UNIT()
);
#59220=SHAPE_DEFINITION_REPRESENTATION(#59241,#59307);
#59241=PRODUCT_DEFINITION_SHAPE('',$,#59329);
#59307=SHAPE_REPRESENTATION('',(#23720),#59194);
#59317=PRODUCT_DEFINITION_CONTEXT('part definition',#59382,'design');
#59329=PRODUCT_DEFINITION('2026-10-23-00-48-09-036',
'01_Front_Housing_Pump_Casing_D100_Flange_D140',#59350,#59317);
#59350=PRODUCT_DEFINITION_FORMATION('',$,#59395);
#59382=APPLICATION_CONTEXT(
'Core Data for Automotive Mechanical Design Process');
#59383=PRODUCT_CONTEXT('part definition',#59382,'mechanical');
#59395=PRODUCT('2026-10-23-00-48-09-036',
'01_Front_Housing_Pump_Casing_D100_Flange_D140',$,(#59383));
#59559=COLOUR_RGB('Dark Blue',0.08,0.2,0.34);
#59560=FILL_AREA_STYLE_COLOUR('',#59559);
#59561=FILL_AREA_STYLE('',(#59560));
#59562=SURFACE_STYLE_FILL_AREA(#59561);
#59563=SURFACE_SIDE_STYLE('',(#59562));
#59564=SURFACE_STYLE_USAGE(.BOTH.,#59563);
#59565=PRESENTATION_STYLE_ASSIGNMENT((#59564));
ENDSEC;
END-ISO-10303-21;
